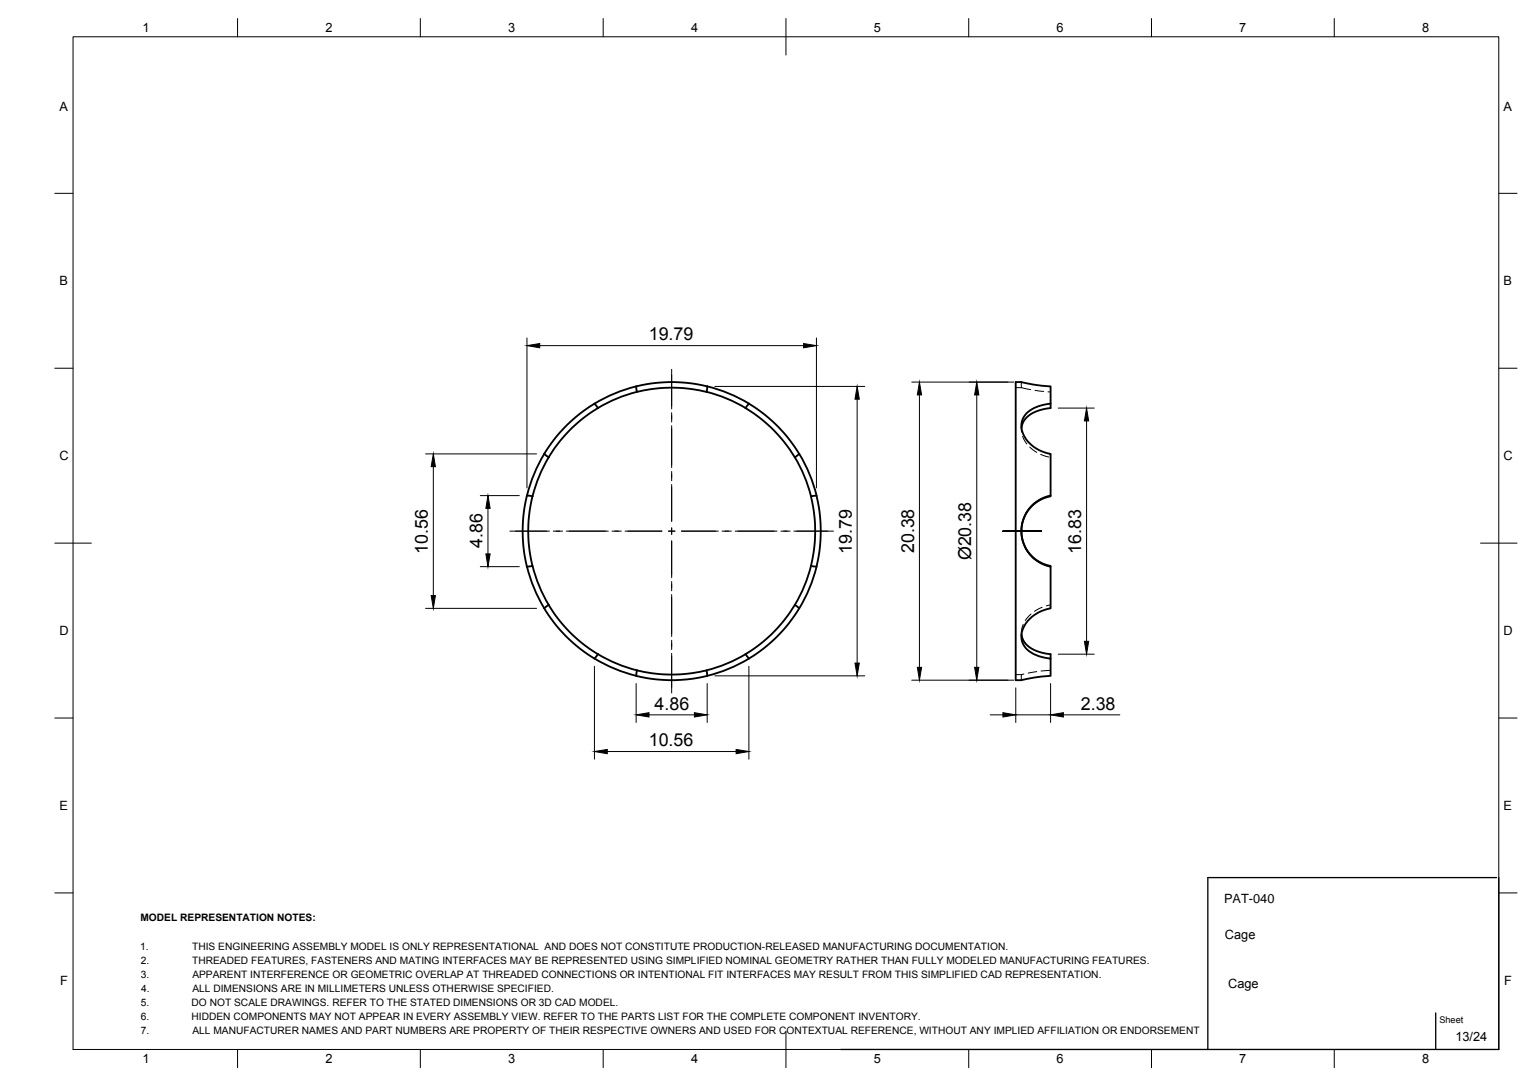
ISO-10303-21;
HEADER;
/* Generated by software containing ST-Developer
 * from STEP Tools, Inc. (www.steptools.com) 
 */

FILE_DESCRIPTION(
/* description */ ('Four-bar tabletop demonstrator'),
/* implementation_level */ '2;1');

FILE_NAME(
/* name */ 'Cage.step',
/* time_stamp */ '2026-10-29T17:05:23-07:00',
/* author */ (''),
/* organization */ (''),
/* preprocessor_version */ 'ST-DEVELOPER v20.2',
/* originating_system */ 'Autodesk Translation Framework v15.17.0.0',
/* authorisation */ '');

FILE_SCHEMA (('AUTOMOTIVE_DESIGN { 1 0 10303 214 3 1 1 }'));
ENDSEC;

DATA;
#10=MECHANICAL_DESIGN_GEOMETRIC_PRESENTATION_REPRESENTATION('',(#351),#6705);
#255=SPHERICAL_SURFACE('',#3806,0.247676);
#256=SPHERICAL_SURFACE('',#3822,0.247676);
#257=SPHERICAL_SURFACE('',#3827,0.247676);
#258=SPHERICAL_SURFACE('',#3832,0.247676);
#259=SPHERICAL_SURFACE('',#3837,0.247676);
#260=SPHERICAL_SURFACE('',#3842,0.247676);
#261=SPHERICAL_SURFACE('',#3847,0.247676);
#262=SPHERICAL_SURFACE('',#3855,0.247676);
#284=B_SPLINE_CURVE_WITH_KNOTS('',3,(#5773,#5774,#5775,#5776,#5777,#5778,
#5779,#5780,#5781,#5782,#5783,#5784,#5785,#5786,#5787,#5788,#5789,#5790,
#5791,#5792,#5793,#5794),.UNSPECIFIED.,.F.,.F.,(4,2,2,2,2,2,2,2,2,2,4),
(0.0473477652366656,0.126350602536658,0.189525903804987,0.252701205073317,
0.313298422430275,0.373895639787233,0.434492857144191,0.495090074501149,
0.558265375769478,0.621440677037807,0.7004435143378),.UNSPECIFIED.);
#285=B_SPLINE_CURVE_WITH_KNOTS('',3,(#5798,#5799,#5800,#5801,#5802,#5803,
#5804,#5805,#5806,#5807,#5808,#5809,#5810,#5811,#5812,#5813,#5814,#5815,
#5816,#5817,#5818,#5819),.UNSPECIFIED.,.F.,.F.,(4,2,2,2,2,2,2,2,2,2,4),
(0.0464897534940957,0.0852567806515119,0.170513561303024,0.246687263103517,
0.308657850341199,0.370628437578881,0.432599024816563,0.494569612054245,
0.570743313854739,0.656000094506251,0.694767121663666),.UNSPECIFIED.);
#286=B_SPLINE_CURVE_WITH_KNOTS('',3,(#5825,#5826,#5827,#5828,#5829,#5830,
#5831,#5832,#5833,#5834,#5835,#5836,#5837,#5838,#5839,#5840,#5841,#5842,
#5843,#5844,#5845,#5846),.UNSPECIFIED.,.F.,.F.,(4,2,2,2,2,2,2,2,2,2,4),
(0.0464897534940957,0.0852567806515118,0.170513561303024,0.246687263103517,
0.308657850341199,0.370628437578881,0.432599024816563,0.494569612054245,
0.570743313854738,0.65600009450625,0.694767121663666),.UNSPECIFIED.);
#287=B_SPLINE_CURVE_WITH_KNOTS('',3,(#5850,#5851,#5852,#5853,#5854,#5855,
#5856,#5857,#5858,#5859,#5860,#5861,#5862,#5863,#5864,#5865,#5866,#5867,
#5868,#5869,#5870,#5871),.UNSPECIFIED.,.F.,.F.,(4,2,2,2,2,2,2,2,2,2,4),
(0.0464897534940957,0.0852567806515119,0.170513561303024,0.246687263103517,
0.308657850341199,0.370628437578881,0.432599024816563,0.494569612054245,
0.570743313854739,0.656000094506251,0.694767121663666),.UNSPECIFIED.);
#288=B_SPLINE_CURVE_WITH_KNOTS('',3,(#5875,#5876,#5877,#5878,#5879,#5880,
#5881,#5882,#5883,#5884,#5885,#5886),.UNSPECIFIED.,.F.,.F.,(4,2,2,2,2,4),
(0.0464897534940957,0.0852567806515119,0.170513561303024,0.246687263103517,
0.308657850341199,0.370628437578881),.UNSPECIFIED.);
#289=B_SPLINE_CURVE_WITH_KNOTS('',3,(#5891,#5892,#5893,#5894,#5895,#5896,
#5897,#5898,#5899,#5900,#5901,#5902),.UNSPECIFIED.,.F.,.F.,(4,2,2,2,2,4),
(0.370628437578881,0.432599024816563,0.494569612054245,0.570743313854738,
0.65600009450625,0.694767121663666),.UNSPECIFIED.);
#290=B_SPLINE_CURVE_WITH_KNOTS('',3,(#5906,#5907,#5908,#5909,#5910,#5911,
#5912,#5913,#5914,#5915,#5916,#5917,#5918,#5919,#5920,#5921,#5922,#5923,
#5924,#5925,#5926,#5927),.UNSPECIFIED.,.F.,.F.,(4,2,2,2,2,2,2,2,2,2,4),
(0.0464897534940957,0.0852567806515121,0.170513561303024,0.246687263103518,
0.308657850341199,0.370628437578881,0.432599024816563,0.494569612054245,
0.570743313854738,0.65600009450625,0.694767121663666),.UNSPECIFIED.);
#291=B_SPLINE_CURVE_WITH_KNOTS('',3,(#5931,#5932,#5933,#5934,#5935,#5936,
#5937,#5938,#5939,#5940,#5941,#5942,#5943,#5944,#5945,#5946,#5947,#5948,
#5949,#5950,#5951,#5952),.UNSPECIFIED.,.F.,.F.,(4,2,2,2,2,2,2,2,2,2,4),
(0.0464897534940957,0.0852567806515119,0.170513561303024,0.246687263103517,
0.308657850341199,0.370628437578881,0.432599024816563,0.494569612054245,
0.570743313854738,0.65600009450625,0.694767121663667),.UNSPECIFIED.);
#292=B_SPLINE_CURVE_WITH_KNOTS('',3,(#5956,#5957,#5958,#5959,#5960,#5961,
#5962,#5963,#5964,#5965,#5966,#5967,#5968,#5969,#5970,#5971,#5972,#5973,
#5974,#5975,#5976,#5977),.UNSPECIFIED.,.F.,.F.,(4,2,2,2,2,2,2,2,2,2,4),
(0.0464897534940957,0.0852567806515119,0.170513561303024,0.246687263103517,
0.308657850341199,0.370628437578881,0.432599024816563,0.494569612054245,
0.570743313854738,0.65600009450625,0.694767121663666),.UNSPECIFIED.);
#293=B_SPLINE_CURVE_WITH_KNOTS('',3,(#5981,#5982,#5983,#5984,#5985,#5986,
#5987,#5988,#5989,#5990,#5991,#5992,#5993,#5994,#5995,#5996,#5997,#5998,
#5999,#6000,#6001,#6002),.UNSPECIFIED.,.F.,.F.,(4,2,2,2,2,2,2,2,2,2,4),
(0.0464897534940957,0.0852567806515119,0.170513561303024,0.246687263103517,
0.308657850341199,0.370628437578881,0.432599024816563,0.494569612054245,
0.570743313854739,0.656000094506251,0.694767121663667),.UNSPECIFIED.);
#294=B_SPLINE_CURVE_WITH_KNOTS('',3,(#6010,#6011,#6012,#6013,#6014,#6015,
#6016,#6017,#6018,#6019,#6020,#6021,#6022,#6023,#6024,#6025,#6026,#6027,
#6028,#6029,#6030,#6031),.UNSPECIFIED.,.F.,.F.,(4,2,2,2,2,2,2,2,2,2,4),
(0.0473477652366656,0.126350602536658,0.189525903804987,0.252701205073316,
0.313298422430274,0.373895639787232,0.434492857144191,0.495090074501149,
0.558265375769478,0.621440677037807,0.7004435143378),.UNSPECIFIED.);
#295=B_SPLINE_CURVE_WITH_KNOTS('',3,(#6039,#6040,#6041,#6042,#6043,#6044,
#6045,#6046,#6047,#6048,#6049,#6050,#6051,#6052,#6053,#6054,#6055,#6056,
#6057,#6058,#6059,#6060),.UNSPECIFIED.,.F.,.F.,(4,2,2,2,2,2,2,2,2,2,4),
(0.0473477652366656,0.126350602536658,0.189525903804987,0.252701205073317,
0.313298422430275,0.373895639787233,0.434492857144191,0.495090074501149,
0.558265375769478,0.621440677037807,0.7004435143378),.UNSPECIFIED.);
#296=B_SPLINE_CURVE_WITH_KNOTS('',3,(#6069,#6070,#6071,#6072,#6073,#6074,
#6075,#6076,#6077,#6078,#6079,#6080),.UNSPECIFIED.,.F.,.F.,(4,2,2,2,2,4),
(0.0473477652366656,0.126350602536658,0.189525903804987,0.252701205073316,
0.313298422430275,0.373895639787233),.UNSPECIFIED.);
#297=B_SPLINE_CURVE_WITH_KNOTS('',3,(#6082,#6083,#6084,#6085,#6086,#6087,
#6088,#6089,#6090,#6091,#6092,#6093),.UNSPECIFIED.,.F.,.F.,(4,2,2,2,2,4),
(0.373895639787233,0.434492857144191,0.495090074501149,0.558265375769478,
0.621440677037807,0.7004435143378),.UNSPECIFIED.);
#298=B_SPLINE_CURVE_WITH_KNOTS('',3,(#6100,#6101,#6102,#6103,#6104,#6105,
#6106,#6107,#6108,#6109,#6110,#6111,#6112,#6113,#6114,#6115,#6116,#6117,
#6118,#6119,#6120,#6121),.UNSPECIFIED.,.F.,.F.,(4,2,2,2,2,2,2,2,2,2,4),
(0.0473477652366656,0.126350602536658,0.189525903804987,0.252701205073316,
0.313298422430275,0.373895639787233,0.434492857144191,0.495090074501149,
0.558265375769478,0.621440677037807,0.7004435143378),.UNSPECIFIED.);
#299=B_SPLINE_CURVE_WITH_KNOTS('',3,(#6129,#6130,#6131,#6132,#6133,#6134,
#6135,#6136,#6137,#6138,#6139,#6140,#6141,#6142,#6143,#6144,#6145,#6146,
#6147,#6148,#6149,#6150),.UNSPECIFIED.,.F.,.F.,(4,2,2,2,2,2,2,2,2,2,4),
(0.0473477652366656,0.126350602536658,0.189525903804987,0.252701205073317,
0.313298422430275,0.373895639787233,0.434492857144191,0.495090074501149,
0.558265375769478,0.621440677037807,0.7004435143378),.UNSPECIFIED.);
#300=B_SPLINE_CURVE_WITH_KNOTS('',3,(#6158,#6159,#6160,#6161,#6162,#6163,
#6164,#6165,#6166,#6167,#6168,#6169,#6170,#6171,#6172,#6173,#6174,#6175,
#6176,#6177,#6178,#6179),.UNSPECIFIED.,.F.,.F.,(4,2,2,2,2,2,2,2,2,2,4),
(0.0473477652366656,0.126350602536658,0.189525903804987,0.252701205073316,
0.313298422430275,0.373895639787233,0.434492857144191,0.495090074501149,
0.558265375769478,0.621440677037807,0.7004435143378),.UNSPECIFIED.);
#301=B_SPLINE_CURVE_WITH_KNOTS('',3,(#6188,#6189,#6190,#6191,#6192,#6193,
#6194,#6195,#6196,#6197,#6198,#6199,#6200,#6201,#6202,#6203,#6204,#6205,
#6206,#6207,#6208,#6209),.UNSPECIFIED.,.F.,.F.,(4,2,2,2,2,2,2,2,2,2,4),
(0.0473477652366656,0.126350602536658,0.189525903804987,0.252701205073317,
0.313298422430275,0.373895639787233,0.434492857144191,0.495090074501149,
0.558265375769478,0.621440677037807,0.7004435143378),.UNSPECIFIED.);
#314=SHAPE_REPRESENTATION_RELATIONSHIP('SRR','None',#6823,#329);
#329=ADVANCED_BREP_SHAPE_REPRESENTATION('',(#373),#6696);
#351=STYLED_ITEM('',(#6989),#373);
#373=MANIFOLD_SOLID_BREP('Continuous crown cage',#3396);
#430=FACE_BOUND('',#938,.T.);
#508=PLANE('',#3819);
#509=PLANE('',#3824);
#510=PLANE('',#3829);
#511=PLANE('',#3834);
#512=PLANE('',#3839);
#513=PLANE('',#3844);
#514=PLANE('',#3853);
#515=PLANE('',#3857);
#516=PLANE('',#3858);
#668=FACE_OUTER_BOUND('',#920,.T.);
#669=FACE_OUTER_BOUND('',#921,.T.);
#670=FACE_OUTER_BOUND('',#922,.T.);
#671=FACE_OUTER_BOUND('',#923,.T.);
#672=FACE_OUTER_BOUND('',#924,.T.);
#673=FACE_OUTER_BOUND('',#925,.T.);
#674=FACE_OUTER_BOUND('',#926,.T.);
#675=FACE_OUTER_BOUND('',#927,.T.);
#676=FACE_OUTER_BOUND('',#928,.T.);
#677=FACE_OUTER_BOUND('',#929,.T.);
#678=FACE_OUTER_BOUND('',#930,.T.);
#679=FACE_OUTER_BOUND('',#931,.T.);
#680=FACE_OUTER_BOUND('',#932,.T.);
#681=FACE_OUTER_BOUND('',#933,.T.);
#682=FACE_OUTER_BOUND('',#934,.T.);
#683=FACE_OUTER_BOUND('',#935,.T.);
#684=FACE_OUTER_BOUND('',#936,.T.);
#685=FACE_OUTER_BOUND('',#937,.T.);
#686=FACE_OUTER_BOUND('',#939,.T.);
#920=EDGE_LOOP('',(#2708,#2709,#2710,#2711));
#921=EDGE_LOOP('',(#2712,#2713,#2714,#2715,#2716,#2717,#2718,#2719,#2720,
#2721,#2722,#2723,#2724,#2725,#2726,#2727,#2728,#2729,#2730,#2731));
#922=EDGE_LOOP('',(#2732,#2733,#2734,#2735));
#923=EDGE_LOOP('',(#2736,#2737,#2738,#2739));
#924=EDGE_LOOP('',(#2740,#2741,#2742,#2743));
#925=EDGE_LOOP('',(#2744,#2745,#2746,#2747));
#926=EDGE_LOOP('',(#2748,#2749,#2750,#2751));
#927=EDGE_LOOP('',(#2752,#2753,#2754,#2755,#2756,#2757));
#928=EDGE_LOOP('',(#2758,#2759,#2760,#2761));
#929=EDGE_LOOP('',(#2762,#2763,#2764,#2765));
#930=EDGE_LOOP('',(#2766,#2767,#2768,#2769));
#931=EDGE_LOOP('',(#2770,#2771,#2772,#2773));
#932=EDGE_LOOP('',(#2774,#2775,#2776,#2777));
#933=EDGE_LOOP('',(#2778,#2779,#2780,#2781));
#934=EDGE_LOOP('',(#2782,#2783,#2784,#2785,#2786,#2787,#2788,#2789,#2790,
#2791,#2792,#2793,#2794,#2795,#2796,#2797,#2798,#2799,#2800,#2801));
#935=EDGE_LOOP('',(#2802,#2803,#2804,#2805));
#936=EDGE_LOOP('',(#2806,#2807,#2808,#2809));
#937=EDGE_LOOP('',(#2810));
#938=EDGE_LOOP('',(#2811));
#939=EDGE_LOOP('',(#2812,#2813,#2814,#2815));
#1140=LINE('',#5888,#1310);
#1141=LINE('',#6184,#1311);
#1310=VECTOR('',#4639,1.019052);
#1311=VECTOR('',#4716,0.980948);
#1504=CIRCLE('',#3807,0.243053047864041);
#1505=CIRCLE('',#3808,0.243053047864041);
#1506=CIRCLE('',#3810,1.019052);
#1507=CIRCLE('',#3811,1.019052);
#1508=CIRCLE('',#3812,1.019052);
#1509=CIRCLE('',#3813,1.019052);
#1510=CIRCLE('',#3814,1.019052);
#1511=CIRCLE('',#3815,1.019052);
#1512=CIRCLE('',#3816,1.019052);
#1513=CIRCLE('',#3817,1.019052);
#1514=CIRCLE('',#3818,1.019052);
#1515=CIRCLE('',#3820,0.980948);
#1516=CIRCLE('',#3821,0.243053047864041);
#1517=CIRCLE('',#3823,0.243053047864041);
#1518=CIRCLE('',#3825,0.980948);
#1519=CIRCLE('',#3826,0.243053047864041);
#1520=CIRCLE('',#3828,0.243053047864041);
#1521=CIRCLE('',#3830,0.980948);
#1522=CIRCLE('',#3831,0.243053047864041);
#1523=CIRCLE('',#3833,0.243053047864041);
#1524=CIRCLE('',#3835,0.980948);
#1525=CIRCLE('',#3836,0.243053047864041);
#1526=CIRCLE('',#3838,0.243053047864041);
#1527=CIRCLE('',#3840,0.980948);
#1528=CIRCLE('',#3841,0.243053047864041);
#1529=CIRCLE('',#3843,0.243053047864041);
#1530=CIRCLE('',#3845,0.980948);
#1531=CIRCLE('',#3846,0.243053047864041);
#1532=CIRCLE('',#3848,0.243053047864041);
#1533=CIRCLE('',#3850,0.980948);
#1534=CIRCLE('',#3851,0.980948);
#1535=CIRCLE('',#3852,0.980948);
#1536=CIRCLE('',#3854,0.243053047864041);
#1537=CIRCLE('',#3856,0.243053047864041);
#1749=VERTEX_POINT('',#5771);
#1750=VERTEX_POINT('',#5772);
#1751=VERTEX_POINT('',#5795);
#1752=VERTEX_POINT('',#5797);
#1753=VERTEX_POINT('',#5822);
#1754=VERTEX_POINT('',#5824);
#1755=VERTEX_POINT('',#5847);
#1756=VERTEX_POINT('',#5849);
#1757=VERTEX_POINT('',#5872);
#1758=VERTEX_POINT('',#5874);
#1759=VERTEX_POINT('',#5887);
#1760=VERTEX_POINT('',#5890);
#1761=VERTEX_POINT('',#5903);
#1762=VERTEX_POINT('',#5905);
#1763=VERTEX_POINT('',#5928);
#1764=VERTEX_POINT('',#5930);
#1765=VERTEX_POINT('',#5953);
#1766=VERTEX_POINT('',#5955);
#1767=VERTEX_POINT('',#5978);
#1768=VERTEX_POINT('',#5980);
#1769=VERTEX_POINT('',#6005);
#1770=VERTEX_POINT('',#6009);
#1771=VERTEX_POINT('',#6034);
#1772=VERTEX_POINT('',#6038);
#1773=VERTEX_POINT('',#6063);
#1774=VERTEX_POINT('',#6067);
#1775=VERTEX_POINT('',#6068);
#1776=VERTEX_POINT('',#6095);
#1777=VERTEX_POINT('',#6099);
#1778=VERTEX_POINT('',#6124);
#1779=VERTEX_POINT('',#6128);
#1780=VERTEX_POINT('',#6153);
#1781=VERTEX_POINT('',#6157);
#1782=VERTEX_POINT('',#6182);
#1783=VERTEX_POINT('',#6185);
#1784=VERTEX_POINT('',#6187);
#2090=EDGE_CURVE('',#1749,#1750,#284,.T.);
#2091=EDGE_CURVE('',#1751,#1749,#1504,.T.);
#2092=EDGE_CURVE('',#1752,#1751,#285,.T.);
#2093=EDGE_CURVE('',#1750,#1752,#1505,.T.);
#2094=EDGE_CURVE('',#1753,#1751,#1506,.T.);
#2095=EDGE_CURVE('',#1753,#1754,#286,.T.);
#2096=EDGE_CURVE('',#1755,#1754,#1507,.T.);
#2097=EDGE_CURVE('',#1755,#1756,#287,.T.);
#2098=EDGE_CURVE('',#1757,#1756,#1508,.T.);
#2099=EDGE_CURVE('',#1757,#1758,#288,.T.);
#2100=EDGE_CURVE('',#1758,#1759,#1140,.T.);
#2101=EDGE_CURVE('',#1759,#1759,#1509,.T.);
#2102=EDGE_CURVE('',#1758,#1760,#289,.T.);
#2103=EDGE_CURVE('',#1761,#1760,#1510,.T.);
#2104=EDGE_CURVE('',#1761,#1762,#290,.T.);
#2105=EDGE_CURVE('',#1763,#1762,#1511,.T.);
#2106=EDGE_CURVE('',#1763,#1764,#291,.T.);
#2107=EDGE_CURVE('',#1765,#1764,#1512,.T.);
#2108=EDGE_CURVE('',#1765,#1766,#292,.T.);
#2109=EDGE_CURVE('',#1767,#1766,#1513,.T.);
#2110=EDGE_CURVE('',#1767,#1768,#293,.T.);
#2111=EDGE_CURVE('',#1752,#1768,#1514,.T.);
#2112=EDGE_CURVE('',#1749,#1769,#1515,.T.);
#2113=EDGE_CURVE('',#1769,#1753,#1516,.T.);
#2114=EDGE_CURVE('',#1770,#1769,#294,.T.);
#2115=EDGE_CURVE('',#1754,#1770,#1517,.T.);
#2116=EDGE_CURVE('',#1770,#1771,#1518,.T.);
#2117=EDGE_CURVE('',#1771,#1755,#1519,.T.);
#2118=EDGE_CURVE('',#1772,#1771,#295,.T.);
#2119=EDGE_CURVE('',#1756,#1772,#1520,.T.);
#2120=EDGE_CURVE('',#1772,#1773,#1521,.T.);
#2121=EDGE_CURVE('',#1773,#1757,#1522,.T.);
#2122=EDGE_CURVE('',#1774,#1775,#296,.T.);
#2123=EDGE_CURVE('',#1760,#1774,#1523,.T.);
#2124=EDGE_CURVE('',#1775,#1773,#297,.T.);
#2125=EDGE_CURVE('',#1774,#1776,#1524,.T.);
#2126=EDGE_CURVE('',#1776,#1761,#1525,.T.);
#2127=EDGE_CURVE('',#1777,#1776,#298,.T.);
#2128=EDGE_CURVE('',#1762,#1777,#1526,.T.);
#2129=EDGE_CURVE('',#1777,#1778,#1527,.T.);
#2130=EDGE_CURVE('',#1778,#1763,#1528,.T.);
#2131=EDGE_CURVE('',#1779,#1778,#299,.T.);
#2132=EDGE_CURVE('',#1764,#1779,#1529,.T.);
#2133=EDGE_CURVE('',#1779,#1780,#1530,.T.);
#2134=EDGE_CURVE('',#1780,#1765,#1531,.T.);
#2135=EDGE_CURVE('',#1781,#1780,#300,.T.);
#2136=EDGE_CURVE('',#1766,#1781,#1532,.T.);
#2137=EDGE_CURVE('',#1782,#1782,#1533,.T.);
#2138=EDGE_CURVE('',#1782,#1775,#1141,.T.);
#2139=EDGE_CURVE('',#1783,#1750,#1534,.T.);
#2140=EDGE_CURVE('',#1783,#1784,#301,.T.);
#2141=EDGE_CURVE('',#1781,#1784,#1535,.T.);
#2142=EDGE_CURVE('',#1768,#1783,#1536,.T.);
#2143=EDGE_CURVE('',#1784,#1767,#1537,.T.);
#2708=ORIENTED_EDGE('',*,*,#2090,.F.);
#2709=ORIENTED_EDGE('',*,*,#2091,.F.);
#2710=ORIENTED_EDGE('',*,*,#2092,.F.);
#2711=ORIENTED_EDGE('',*,*,#2093,.F.);
#2712=ORIENTED_EDGE('',*,*,#2092,.T.);
#2713=ORIENTED_EDGE('',*,*,#2094,.F.);
#2714=ORIENTED_EDGE('',*,*,#2095,.T.);
#2715=ORIENTED_EDGE('',*,*,#2096,.F.);
#2716=ORIENTED_EDGE('',*,*,#2097,.T.);
#2717=ORIENTED_EDGE('',*,*,#2098,.F.);
#2718=ORIENTED_EDGE('',*,*,#2099,.T.);
#2719=ORIENTED_EDGE('',*,*,#2100,.T.);
#2720=ORIENTED_EDGE('',*,*,#2101,.F.);
#2721=ORIENTED_EDGE('',*,*,#2100,.F.);
#2722=ORIENTED_EDGE('',*,*,#2102,.T.);
#2723=ORIENTED_EDGE('',*,*,#2103,.F.);
#2724=ORIENTED_EDGE('',*,*,#2104,.T.);
#2725=ORIENTED_EDGE('',*,*,#2105,.F.);
#2726=ORIENTED_EDGE('',*,*,#2106,.T.);
#2727=ORIENTED_EDGE('',*,*,#2107,.F.);
#2728=ORIENTED_EDGE('',*,*,#2108,.T.);
#2729=ORIENTED_EDGE('',*,*,#2109,.F.);
#2730=ORIENTED_EDGE('',*,*,#2110,.T.);
#2731=ORIENTED_EDGE('',*,*,#2111,.F.);
#2732=ORIENTED_EDGE('',*,*,#2091,.T.);
#2733=ORIENTED_EDGE('',*,*,#2112,.T.);
#2734=ORIENTED_EDGE('',*,*,#2113,.T.);
#2735=ORIENTED_EDGE('',*,*,#2094,.T.);
#2736=ORIENTED_EDGE('',*,*,#2114,.F.);
#2737=ORIENTED_EDGE('',*,*,#2115,.F.);
#2738=ORIENTED_EDGE('',*,*,#2095,.F.);
#2739=ORIENTED_EDGE('',*,*,#2113,.F.);
#2740=ORIENTED_EDGE('',*,*,#2115,.T.);
#2741=ORIENTED_EDGE('',*,*,#2116,.T.);
#2742=ORIENTED_EDGE('',*,*,#2117,.T.);
#2743=ORIENTED_EDGE('',*,*,#2096,.T.);
#2744=ORIENTED_EDGE('',*,*,#2118,.F.);
#2745=ORIENTED_EDGE('',*,*,#2119,.F.);
#2746=ORIENTED_EDGE('',*,*,#2097,.F.);
#2747=ORIENTED_EDGE('',*,*,#2117,.F.);
#2748=ORIENTED_EDGE('',*,*,#2119,.T.);
#2749=ORIENTED_EDGE('',*,*,#2120,.T.);
#2750=ORIENTED_EDGE('',*,*,#2121,.T.);
#2751=ORIENTED_EDGE('',*,*,#2098,.T.);
#2752=ORIENTED_EDGE('',*,*,#2122,.F.);
#2753=ORIENTED_EDGE('',*,*,#2123,.F.);
#2754=ORIENTED_EDGE('',*,*,#2102,.F.);
#2755=ORIENTED_EDGE('',*,*,#2099,.F.);
#2756=ORIENTED_EDGE('',*,*,#2121,.F.);
#2757=ORIENTED_EDGE('',*,*,#2124,.F.);
#2758=ORIENTED_EDGE('',*,*,#2123,.T.);
#2759=ORIENTED_EDGE('',*,*,#2125,.T.);
#2760=ORIENTED_EDGE('',*,*,#2126,.T.);
#2761=ORIENTED_EDGE('',*,*,#2103,.T.);
#2762=ORIENTED_EDGE('',*,*,#2127,.F.);
#2763=ORIENTED_EDGE('',*,*,#2128,.F.);
#2764=ORIENTED_EDGE('',*,*,#2104,.F.);
#2765=ORIENTED_EDGE('',*,*,#2126,.F.);
#2766=ORIENTED_EDGE('',*,*,#2128,.T.);
#2767=ORIENTED_EDGE('',*,*,#2129,.T.);
#2768=ORIENTED_EDGE('',*,*,#2130,.T.);
#2769=ORIENTED_EDGE('',*,*,#2105,.T.);
#2770=ORIENTED_EDGE('',*,*,#2131,.F.);
#2771=ORIENTED_EDGE('',*,*,#2132,.F.);
#2772=ORIENTED_EDGE('',*,*,#2106,.F.);
#2773=ORIENTED_EDGE('',*,*,#2130,.F.);
#2774=ORIENTED_EDGE('',*,*,#2132,.T.);
#2775=ORIENTED_EDGE('',*,*,#2133,.T.);
#2776=ORIENTED_EDGE('',*,*,#2134,.T.);
#2777=ORIENTED_EDGE('',*,*,#2107,.T.);
#2778=ORIENTED_EDGE('',*,*,#2108,.F.);
#2779=ORIENTED_EDGE('',*,*,#2134,.F.);
#2780=ORIENTED_EDGE('',*,*,#2135,.F.);
#2781=ORIENTED_EDGE('',*,*,#2136,.F.);
#2782=ORIENTED_EDGE('',*,*,#2137,.F.);
#2783=ORIENTED_EDGE('',*,*,#2138,.T.);
#2784=ORIENTED_EDGE('',*,*,#2124,.T.);
#2785=ORIENTED_EDGE('',*,*,#2120,.F.);
#2786=ORIENTED_EDGE('',*,*,#2118,.T.);
#2787=ORIENTED_EDGE('',*,*,#2116,.F.);
#2788=ORIENTED_EDGE('',*,*,#2114,.T.);
#2789=ORIENTED_EDGE('',*,*,#2112,.F.);
#2790=ORIENTED_EDGE('',*,*,#2090,.T.);
#2791=ORIENTED_EDGE('',*,*,#2139,.F.);
#2792=ORIENTED_EDGE('',*,*,#2140,.T.);
#2793=ORIENTED_EDGE('',*,*,#2141,.F.);
#2794=ORIENTED_EDGE('',*,*,#2135,.T.);
#2795=ORIENTED_EDGE('',*,*,#2133,.F.);
#2796=ORIENTED_EDGE('',*,*,#2131,.T.);
#2797=ORIENTED_EDGE('',*,*,#2129,.F.);
#2798=ORIENTED_EDGE('',*,*,#2127,.T.);
#2799=ORIENTED_EDGE('',*,*,#2125,.F.);
#2800=ORIENTED_EDGE('',*,*,#2122,.T.);
#2801=ORIENTED_EDGE('',*,*,#2138,.F.);
#2802=ORIENTED_EDGE('',*,*,#2093,.T.);
#2803=ORIENTED_EDGE('',*,*,#2111,.T.);
#2804=ORIENTED_EDGE('',*,*,#2142,.T.);
#2805=ORIENTED_EDGE('',*,*,#2139,.T.);
#2806=ORIENTED_EDGE('',*,*,#2110,.F.);
#2807=ORIENTED_EDGE('',*,*,#2143,.F.);
#2808=ORIENTED_EDGE('',*,*,#2140,.F.);
#2809=ORIENTED_EDGE('',*,*,#2142,.F.);
#2810=ORIENTED_EDGE('',*,*,#2101,.T.);
#2811=ORIENTED_EDGE('',*,*,#2137,.T.);
#2812=ORIENTED_EDGE('',*,*,#2136,.T.);
#2813=ORIENTED_EDGE('',*,*,#2141,.T.);
#2814=ORIENTED_EDGE('',*,*,#2143,.T.);
#2815=ORIENTED_EDGE('',*,*,#2109,.T.);
#3147=CYLINDRICAL_SURFACE('',#3809,1.019052);
#3148=CYLINDRICAL_SURFACE('',#3849,0.980948);
#3284=ADVANCED_FACE('',(#668),#255,.F.);
#3285=ADVANCED_FACE('',(#669),#3147,.T.);
#3286=ADVANCED_FACE('',(#670),#508,.T.);
#3287=ADVANCED_FACE('',(#671),#256,.F.);
#3288=ADVANCED_FACE('',(#672),#509,.T.);
#3289=ADVANCED_FACE('',(#673),#257,.F.);
#3290=ADVANCED_FACE('',(#674),#510,.T.);
#3291=ADVANCED_FACE('',(#675),#258,.F.);
#3292=ADVANCED_FACE('',(#676),#511,.T.);
#3293=ADVANCED_FACE('',(#677),#259,.F.);
#3294=ADVANCED_FACE('',(#678),#512,.T.);
#3295=ADVANCED_FACE('',(#679),#260,.F.);
#3296=ADVANCED_FACE('',(#680),#513,.T.);
#3297=ADVANCED_FACE('',(#681),#261,.F.);
#3298=ADVANCED_FACE('',(#682),#3148,.F.);
#3299=ADVANCED_FACE('',(#683),#514,.T.);
#3300=ADVANCED_FACE('',(#684),#262,.F.);
#3301=ADVANCED_FACE('',(#685,#430),#515,.T.);
#3302=ADVANCED_FACE('',(#686),#516,.T.);
#3396=CLOSED_SHELL('',(#3284,#3285,#3286,#3287,#3288,#3289,#3290,#3291,
#3292,#3293,#3294,#3295,#3296,#3297,#3298,#3299,#3300,#3301,#3302));
#3805=AXIS2_PLACEMENT_3D('',#5769,#4623,#4624);
#3806=AXIS2_PLACEMENT_3D('',#5770,#4625,#4626);
#3807=AXIS2_PLACEMENT_3D('',#5796,#4627,#4628);
#3808=AXIS2_PLACEMENT_3D('',#5820,#4629,#4630);
#3809=AXIS2_PLACEMENT_3D('',#5821,#4631,#4632);
#3810=AXIS2_PLACEMENT_3D('',#5823,#4633,#4634);
#3811=AXIS2_PLACEMENT_3D('',#5848,#4635,#4636);
#3812=AXIS2_PLACEMENT_3D('',#5873,#4637,#4638);
#3813=AXIS2_PLACEMENT_3D('',#5889,#4640,#4641);
#3814=AXIS2_PLACEMENT_3D('',#5904,#4642,#4643);
#3815=AXIS2_PLACEMENT_3D('',#5929,#4644,#4645);
#3816=AXIS2_PLACEMENT_3D('',#5954,#4646,#4647);
#3817=AXIS2_PLACEMENT_3D('',#5979,#4648,#4649);
#3818=AXIS2_PLACEMENT_3D('',#6003,#4650,#4651);
#3819=AXIS2_PLACEMENT_3D('',#6004,#4652,#4653);
#3820=AXIS2_PLACEMENT_3D('',#6006,#4654,#4655);
#3821=AXIS2_PLACEMENT_3D('',#6007,#4656,#4657);
#3822=AXIS2_PLACEMENT_3D('',#6008,#4658,#4659);
#3823=AXIS2_PLACEMENT_3D('',#6032,#4660,#4661);
#3824=AXIS2_PLACEMENT_3D('',#6033,#4662,#4663);
#3825=AXIS2_PLACEMENT_3D('',#6035,#4664,#4665);
#3826=AXIS2_PLACEMENT_3D('',#6036,#4666,#4667);
#3827=AXIS2_PLACEMENT_3D('',#6037,#4668,#4669);
#3828=AXIS2_PLACEMENT_3D('',#6061,#4670,#4671);
#3829=AXIS2_PLACEMENT_3D('',#6062,#4672,#4673);
#3830=AXIS2_PLACEMENT_3D('',#6064,#4674,#4675);
#3831=AXIS2_PLACEMENT_3D('',#6065,#4676,#4677);
#3832=AXIS2_PLACEMENT_3D('',#6066,#4678,#4679);
#3833=AXIS2_PLACEMENT_3D('',#6081,#4680,#4681);
#3834=AXIS2_PLACEMENT_3D('',#6094,#4682,#4683);
#3835=AXIS2_PLACEMENT_3D('',#6096,#4684,#4685);
#3836=AXIS2_PLACEMENT_3D('',#6097,#4686,#4687);
#3837=AXIS2_PLACEMENT_3D('',#6098,#4688,#4689);
#3838=AXIS2_PLACEMENT_3D('',#6122,#4690,#4691);
#3839=AXIS2_PLACEMENT_3D('',#6123,#4692,#4693);
#3840=AXIS2_PLACEMENT_3D('',#6125,#4694,#4695);
#3841=AXIS2_PLACEMENT_3D('',#6126,#4696,#4697);
#3842=AXIS2_PLACEMENT_3D('',#6127,#4698,#4699);
#3843=AXIS2_PLACEMENT_3D('',#6151,#4700,#4701);
#3844=AXIS2_PLACEMENT_3D('',#6152,#4702,#4703);
#3845=AXIS2_PLACEMENT_3D('',#6154,#4704,#4705);
#3846=AXIS2_PLACEMENT_3D('',#6155,#4706,#4707);
#3847=AXIS2_PLACEMENT_3D('',#6156,#4708,#4709);
#3848=AXIS2_PLACEMENT_3D('',#6180,#4710,#4711);
#3849=AXIS2_PLACEMENT_3D('',#6181,#4712,#4713);
#3850=AXIS2_PLACEMENT_3D('',#6183,#4714,#4715);
#3851=AXIS2_PLACEMENT_3D('',#6186,#4717,#4718);
#3852=AXIS2_PLACEMENT_3D('',#6210,#4719,#4720);
#3853=AXIS2_PLACEMENT_3D('',#6211,#4721,#4722);
#3854=AXIS2_PLACEMENT_3D('',#6212,#4723,#4724);
#3855=AXIS2_PLACEMENT_3D('',#6213,#4725,#4726);
#3856=AXIS2_PLACEMENT_3D('',#6214,#4727,#4728);
#3857=AXIS2_PLACEMENT_3D('',#6215,#4729,#4730);
#3858=AXIS2_PLACEMENT_3D('',#6216,#4731,#4732);
#4623=DIRECTION('axis',(0.,0.,1.));
#4624=DIRECTION('refdir',(1.,0.,0.));
#4625=DIRECTION('center_axis',(0.,0.,1.));
#4626=DIRECTION('ref_axis',(1.,0.,0.));
#4627=DIRECTION('center_axis',(0.,-1.,0.));
#4628=DIRECTION('ref_axis',(0.,0.,-1.));
#4629=DIRECTION('center_axis',(0.,-1.,0.));
#4630=DIRECTION('ref_axis',(0.,0.,-1.));
#4631=DIRECTION('center_axis',(0.,1.,0.));
#4632=DIRECTION('ref_axis',(1.,0.,0.));
#4633=DIRECTION('center_axis',(0.,1.,0.));
#4634=DIRECTION('ref_axis',(1.,0.,0.));
#4635=DIRECTION('center_axis',(0.,1.,0.));
#4636=DIRECTION('ref_axis',(1.,0.,0.));
#4637=DIRECTION('center_axis',(0.,1.,0.));
#4638=DIRECTION('ref_axis',(1.,0.,0.));
#4639=DIRECTION('',(0.,-1.,0.));
#4640=DIRECTION('center_axis',(0.,-1.,0.));
#4641=DIRECTION('ref_axis',(1.,0.,0.));
#4642=DIRECTION('center_axis',(0.,1.,0.));
#4643=DIRECTION('ref_axis',(1.,0.,0.));
#4644=DIRECTION('center_axis',(0.,1.,0.));
#4645=DIRECTION('ref_axis',(1.,0.,0.));
#4646=DIRECTION('center_axis',(0.,1.,0.));
#4647=DIRECTION('ref_axis',(1.,0.,0.));
#4648=DIRECTION('center_axis',(0.,1.,0.));
#4649=DIRECTION('ref_axis',(1.,0.,0.));
#4650=DIRECTION('center_axis',(0.,1.,0.));
#4651=DIRECTION('ref_axis',(1.,0.,0.));
#4652=DIRECTION('center_axis',(0.,1.,0.));
#4653=DIRECTION('ref_axis',(1.,0.,0.));
#4654=DIRECTION('center_axis',(0.,-1.,0.));
#4655=DIRECTION('ref_axis',(1.,0.,0.));
#4656=DIRECTION('center_axis',(0.,-1.,0.));
#4657=DIRECTION('ref_axis',(0.,0.,-1.));
#4658=DIRECTION('center_axis',(6.12323399573677E-17,0.,1.));
#4659=DIRECTION('ref_axis',(1.,0.,0.));
#4660=DIRECTION('center_axis',(0.,-1.,0.));
#4661=DIRECTION('ref_axis',(0.,0.,-1.));
#4662=DIRECTION('center_axis',(0.,1.,0.));
#4663=DIRECTION('ref_axis',(1.,0.,0.));
#4664=DIRECTION('center_axis',(0.,-1.,0.));
#4665=DIRECTION('ref_axis',(1.,0.,0.));
#4666=DIRECTION('center_axis',(0.,-1.,0.));
#4667=DIRECTION('ref_axis',(0.,0.,-1.));
#4668=DIRECTION('center_axis',(0.,0.,1.));
#4669=DIRECTION('ref_axis',(1.,0.,0.));
#4670=DIRECTION('center_axis',(0.,-1.,0.));
#4671=DIRECTION('ref_axis',(0.,0.,-1.));
#4672=DIRECTION('center_axis',(0.,1.,0.));
#4673=DIRECTION('ref_axis',(1.,0.,0.));
#4674=DIRECTION('center_axis',(0.,-1.,0.));
#4675=DIRECTION('ref_axis',(1.,0.,0.));
#4676=DIRECTION('center_axis',(0.,-1.,0.));
#4677=DIRECTION('ref_axis',(0.,0.,-1.));
#4678=DIRECTION('center_axis',(0.,0.,1.));
#4679=DIRECTION('ref_axis',(1.,0.,0.));
#4680=DIRECTION('center_axis',(0.,-1.,0.));
#4681=DIRECTION('ref_axis',(0.,0.,-1.));
#4682=DIRECTION('center_axis',(0.,1.,0.));
#4683=DIRECTION('ref_axis',(1.,0.,0.));
#4684=DIRECTION('center_axis',(0.,-1.,0.));
#4685=DIRECTION('ref_axis',(1.,0.,0.));
#4686=DIRECTION('center_axis',(0.,-1.,0.));
#4687=DIRECTION('ref_axis',(0.,0.,-1.));
#4688=DIRECTION('center_axis',(0.,0.,1.));
#4689=DIRECTION('ref_axis',(1.,0.,0.));
#4690=DIRECTION('center_axis',(0.,-1.,0.));
#4691=DIRECTION('ref_axis',(0.,0.,-1.));
#4692=DIRECTION('center_axis',(0.,1.,0.));
#4693=DIRECTION('ref_axis',(1.,0.,0.));
#4694=DIRECTION('center_axis',(0.,-1.,0.));
#4695=DIRECTION('ref_axis',(1.,0.,0.));
#4696=DIRECTION('center_axis',(0.,-1.,0.));
#4697=DIRECTION('ref_axis',(0.,0.,-1.));
#4698=DIRECTION('center_axis',(6.12323399573676E-17,0.,1.));
#4699=DIRECTION('ref_axis',(1.,0.,0.));
#4700=DIRECTION('center_axis',(0.,-1.,0.));
#4701=DIRECTION('ref_axis',(0.,0.,-1.));
#4702=DIRECTION('center_axis',(0.,1.,0.));
#4703=DIRECTION('ref_axis',(1.,0.,0.));
#4704=DIRECTION('center_axis',(0.,-1.,0.));
#4705=DIRECTION('ref_axis',(1.,0.,0.));
#4706=DIRECTION('center_axis',(0.,-1.,0.));
#4707=DIRECTION('ref_axis',(0.,0.,-1.));
#4708=DIRECTION('center_axis',(0.,0.,1.));
#4709=DIRECTION('ref_axis',(1.,0.,0.));
#4710=DIRECTION('center_axis',(0.,-1.,0.));
#4711=DIRECTION('ref_axis',(0.,0.,-1.));
#4712=DIRECTION('center_axis',(0.,1.,0.));
#4713=DIRECTION('ref_axis',(1.,0.,0.));
#4714=DIRECTION('center_axis',(0.,1.,0.));
#4715=DIRECTION('ref_axis',(1.,0.,0.));
#4716=DIRECTION('',(0.,1.,0.));
#4717=DIRECTION('center_axis',(0.,-1.,0.));
#4718=DIRECTION('ref_axis',(1.,0.,0.));
#4719=DIRECTION('center_axis',(0.,-1.,0.));
#4720=DIRECTION('ref_axis',(1.,0.,0.));
#4721=DIRECTION('center_axis',(0.,1.,0.));
#4722=DIRECTION('ref_axis',(1.,0.,0.));
#4723=DIRECTION('center_axis',(0.,-1.,0.));
#4724=DIRECTION('ref_axis',(0.,0.,-1.));
#4725=DIRECTION('center_axis',(0.,0.,1.));
#4726=DIRECTION('ref_axis',(1.,0.,0.));
#4727=DIRECTION('center_axis',(0.,-1.,0.));
#4728=DIRECTION('ref_axis',(0.,0.,-1.));
#4729=DIRECTION('center_axis',(0.,-1.,0.));
#4730=DIRECTION('ref_axis',(-1.,0.,0.));
#4731=DIRECTION('center_axis',(0.,1.,0.));
#4732=DIRECTION('ref_axis',(1.,0.,0.));
#5769=CARTESIAN_POINT('',(0.,0.,0.));
#5770=CARTESIAN_POINT('Origin',(0.707106781186547,0.,0.707106781186548));
#5771=CARTESIAN_POINT('',(0.504455939115715,-0.04763,0.841298510752802));
#5772=CARTESIAN_POINT('',(0.841298510752802,-0.04763,0.504455939115715));
#5773=CARTESIAN_POINT('Ctrl Pts',(0.504455939115715,-0.04763,0.841298510752802));
#5774=CARTESIAN_POINT('Ctrl Pts',(0.508899795931835,-0.0740444353928835,
0.838633903678357));
#5775=CARTESIAN_POINT('Ctrl Pts',(0.517157748491652,-0.0999305678883309,
0.833661031856294));
#5776=CARTESIAN_POINT('Ctrl Pts',(0.537715343527944,-0.142345102874864,
0.820511285096538));
#5777=CARTESIAN_POINT('Ctrl Pts',(0.548874290046456,-0.159766064500479,
0.813159949759));
#5778=CARTESIAN_POINT('Ctrl Pts',(0.573915184558107,-0.190326085855194,
0.795684265985089));
#5779=CARTESIAN_POINT('Ctrl Pts',(0.587792702767295,-0.203463743702801,
0.78555112003688));
#5780=CARTESIAN_POINT('Ctrl Pts',(0.615966552324775,-0.224161999508995,
0.763642258217233));
#5781=CARTESIAN_POINT('Ctrl Pts',(0.631684198665438,-0.232861760990032,
0.750785745543687));
#5782=CARTESIAN_POINT('Ctrl Pts',(0.663382628119203,-0.244251601209411,
0.722929908501543));
#5783=CARTESIAN_POINT('Ctrl Pts',(0.679352081686668,-0.246942143572133,
0.707917883896095));
#5784=CARTESIAN_POINT('Ctrl Pts',(0.707917883896095,-0.246942143572133,
0.679352081686668));
#5785=CARTESIAN_POINT('Ctrl Pts',(0.722929908501543,-0.244251601209411,
0.663382628119203));
#5786=CARTESIAN_POINT('Ctrl Pts',(0.750785745543687,-0.232861760990032,
0.631684198665439));
#5787=CARTESIAN_POINT('Ctrl Pts',(0.763642258217232,-0.224161999508995,
0.615966552324775));
#5788=CARTESIAN_POINT('Ctrl Pts',(0.78555112003688,-0.203463743702801,0.587792702767295));
#5789=CARTESIAN_POINT('Ctrl Pts',(0.795684265985088,-0.190326085855194,
0.573915184558108));
#5790=CARTESIAN_POINT('Ctrl Pts',(0.813159949759,-0.15976606450048,0.548874290046456));
#5791=CARTESIAN_POINT('Ctrl Pts',(0.820511285096538,-0.142345102874864,
0.537715343527944));
#5792=CARTESIAN_POINT('Ctrl Pts',(0.833661031856294,-0.099930567888331,
0.517157748491653));
#5793=CARTESIAN_POINT('Ctrl Pts',(0.838633903678357,-0.0740444353928835,
0.508899795931835));
#5794=CARTESIAN_POINT('Ctrl Pts',(0.841298510752801,-0.0476299999999999,
0.504455939115715));
#5795=CARTESIAN_POINT('',(0.528110872004958,-0.04763,0.871530771444223));
#5796=CARTESIAN_POINT('Origin',(0.707106781186547,-0.04763,0.707106781186548));
#5797=CARTESIAN_POINT('',(0.871530771444223,-0.04763,0.528110872004959));
#5798=CARTESIAN_POINT('Ctrl Pts',(0.871530771444223,-0.0476300000000001,
0.528110872004958));
#5799=CARTESIAN_POINT('Ctrl Pts',(0.87014664509073,-0.0609922781173483,
0.530395067942936));
#5800=CARTESIAN_POINT('Ctrl Pts',(0.868149331745851,-0.0742967091364493,
0.533674141594226));
#5801=CARTESIAN_POINT('Ctrl Pts',(0.85981294420286,-0.115492077056649,0.54708917182331));
#5802=CARTESIAN_POINT('Ctrl Pts',(0.850993704737257,-0.141695629206859,
0.560922177770136));
#5803=CARTESIAN_POINT('Ctrl Pts',(0.830754510485543,-0.181890537957859,
0.590422647829571));
#5804=CARTESIAN_POINT('Ctrl Pts',(0.816896541396381,-0.201072148666545,
0.609616703125488));
#5805=CARTESIAN_POINT('Ctrl Pts',(0.792310597819928,-0.223955109275652,
0.641117951819998));
#5806=CARTESIAN_POINT('Ctrl Pts',(0.779109323683612,-0.232742381310829,
0.657208095763053));
#5807=CARTESIAN_POINT('Ctrl Pts',(0.750552691816206,-0.244234834628584,
0.68964083160521));
#5808=CARTESIAN_POINT('Ctrl Pts',(0.735185187071673,-0.246942143572133,
0.705971972091755));
#5809=CARTESIAN_POINT('Ctrl Pts',(0.705971972091754,-0.246942143572133,
0.735185187071673));
#5810=CARTESIAN_POINT('Ctrl Pts',(0.689640831605209,-0.244234834628584,
0.750552691816206));
#5811=CARTESIAN_POINT('Ctrl Pts',(0.657208095763052,-0.232742381310829,
0.779109323683612));
#5812=CARTESIAN_POINT('Ctrl Pts',(0.641117951819998,-0.223955109275652,
0.792310597819928));
#5813=CARTESIAN_POINT('Ctrl Pts',(0.609616703125487,-0.201072148666545,
0.816896541396382));
#5814=CARTESIAN_POINT('Ctrl Pts',(0.590422647829571,-0.181890537957858,
0.830754510485544));
#5815=CARTESIAN_POINT('Ctrl Pts',(0.560922177770135,-0.141695629206858,
0.850993704737257));
#5816=CARTESIAN_POINT('Ctrl Pts',(0.547089171823309,-0.115492077056649,
0.859812944202861));
#5817=CARTESIAN_POINT('Ctrl Pts',(0.533674141594226,-0.0742967091364491,
0.868149331745852));
#5818=CARTESIAN_POINT('Ctrl Pts',(0.530395067942936,-0.0609922781173483,
0.870146645090731));
#5819=CARTESIAN_POINT('Ctrl Pts',(0.528110872004958,-0.0476300000000001,
0.871530771444223));
#5820=CARTESIAN_POINT('Origin',(0.707106781186547,-0.04763,0.707106781186548));
#5821=CARTESIAN_POINT('Origin',(0.,-0.166705,0.));
#5822=CARTESIAN_POINT('',(0.242834539687906,-0.04763,0.989696097314));
#5823=CARTESIAN_POINT('Origin',(0.,-0.04763,0.));
#5824=CARTESIAN_POINT('',(-0.242834539687907,-0.04763,0.989696097314));
#5825=CARTESIAN_POINT('Ctrl Pts',(0.242834539687906,-0.04763,0.989696097314));
#5826=CARTESIAN_POINT('Ctrl Pts',(0.24024064412003,-0.0609922781173483,
0.990332542620729));
#5827=CARTESIAN_POINT('Ctrl Pts',(0.236509675094874,-0.0742967091364492,
0.991238884025248));
#5828=CARTESIAN_POINT('Ctrl Pts',(0.221129100087819,-0.115492077056649,
0.994830026707808));
#5829=CARTESIAN_POINT('Ctrl Pts',(0.205111543747588,-0.141695629206859,
0.998375294985966));
#5830=CARTESIAN_POINT('Ctrl Pts',(0.169940289819232,-0.181890537957859,
1.00492400591205));
#5831=CARTESIAN_POINT('Ctrl Pts',(0.1465689792446,-0.201072148666545,1.00869718865384));
#5832=CARTESIAN_POINT('Ctrl Pts',(0.106909345252087,-0.223955109275652,
1.01358704779679));
#5833=CARTESIAN_POINT('Ctrl Pts',(0.0861971848975941,-0.232742381310829,
1.0156297872271));
#5834=CARTESIAN_POINT('Ctrl Pts',(0.0430711894098822,-0.244234834628584,
1.01837060663223));
#5835=CARTESIAN_POINT('Ctrl Pts',(0.0206568624125605,-0.246942143572133,
1.019052));
#5836=CARTESIAN_POINT('Ctrl Pts',(-0.0206568624125608,-0.246942143572133,
1.019052));
#5837=CARTESIAN_POINT('Ctrl Pts',(-0.0430711894098825,-0.244234834628584,
1.01837060663223));
#5838=CARTESIAN_POINT('Ctrl Pts',(-0.0861971848975943,-0.232742381310829,
1.0156297872271));
#5839=CARTESIAN_POINT('Ctrl Pts',(-0.106909345252088,-0.223955109275652,
1.01358704779679));
#5840=CARTESIAN_POINT('Ctrl Pts',(-0.1465689792446,-0.201072148666545,1.00869718865384));
#5841=CARTESIAN_POINT('Ctrl Pts',(-0.169940289819232,-0.181890537957859,
1.00492400591205));
#5842=CARTESIAN_POINT('Ctrl Pts',(-0.205111543747588,-0.141695629206859,
0.998375294985966));
#5843=CARTESIAN_POINT('Ctrl Pts',(-0.221129100087819,-0.115492077056649,
0.994830026707808));
#5844=CARTESIAN_POINT('Ctrl Pts',(-0.236509675094875,-0.0742967091364493,
0.991238884025248));
#5845=CARTESIAN_POINT('Ctrl Pts',(-0.24024064412003,-0.0609922781173483,
0.990332542620729));
#5846=CARTESIAN_POINT('Ctrl Pts',(-0.242834539687907,-0.04763,0.989696097314));
#5847=CARTESIAN_POINT('',(-0.528110872004959,-0.04763,0.871530771444223));
#5848=CARTESIAN_POINT('Origin',(0.,-0.04763,0.));
#5849=CARTESIAN_POINT('',(-0.871530771444223,-0.04763,0.528110872004958));
#5850=CARTESIAN_POINT('Ctrl Pts',(-0.528110872004958,-0.0476300000000001,
0.871530771444223));
#5851=CARTESIAN_POINT('Ctrl Pts',(-0.530395067942936,-0.0609922781173484,
0.87014664509073));
#5852=CARTESIAN_POINT('Ctrl Pts',(-0.533674141594226,-0.0742967091364493,
0.868149331745851));
#5853=CARTESIAN_POINT('Ctrl Pts',(-0.54708917182331,-0.115492077056649,
0.85981294420286));
#5854=CARTESIAN_POINT('Ctrl Pts',(-0.560922177770136,-0.141695629206859,
0.850993704737257));
#5855=CARTESIAN_POINT('Ctrl Pts',(-0.590422647829571,-0.181890537957859,
0.830754510485543));
#5856=CARTESIAN_POINT('Ctrl Pts',(-0.609616703125488,-0.201072148666545,
0.816896541396381));
#5857=CARTESIAN_POINT('Ctrl Pts',(-0.641117951819998,-0.223955109275652,
0.792310597819928));
#5858=CARTESIAN_POINT('Ctrl Pts',(-0.657208095763053,-0.232742381310829,
0.779109323683611));
#5859=CARTESIAN_POINT('Ctrl Pts',(-0.68964083160521,-0.244234834628584,
0.750552691816205));
#5860=CARTESIAN_POINT('Ctrl Pts',(-0.705971972091755,-0.246942143572133,
0.735185187071673));
#5861=CARTESIAN_POINT('Ctrl Pts',(-0.735185187071673,-0.246942143572133,
0.705971972091754));
#5862=CARTESIAN_POINT('Ctrl Pts',(-0.750552691816206,-0.244234834628584,
0.689640831605209));
#5863=CARTESIAN_POINT('Ctrl Pts',(-0.779109323683612,-0.232742381310829,
0.657208095763052));
#5864=CARTESIAN_POINT('Ctrl Pts',(-0.792310597819928,-0.223955109275652,
0.641117951819998));
#5865=CARTESIAN_POINT('Ctrl Pts',(-0.816896541396382,-0.201072148666545,
0.609616703125487));
#5866=CARTESIAN_POINT('Ctrl Pts',(-0.830754510485544,-0.181890537957858,
0.590422647829571));
#5867=CARTESIAN_POINT('Ctrl Pts',(-0.850993704737257,-0.141695629206858,
0.560922177770135));
#5868=CARTESIAN_POINT('Ctrl Pts',(-0.859812944202861,-0.115492077056649,
0.547089171823309));
#5869=CARTESIAN_POINT('Ctrl Pts',(-0.868149331745852,-0.0742967091364491,
0.533674141594226));
#5870=CARTESIAN_POINT('Ctrl Pts',(-0.870146645090731,-0.0609922781173483,
0.530395067942936));
#5871=CARTESIAN_POINT('Ctrl Pts',(-0.871530771444223,-0.04763,0.528110872004958));
#5872=CARTESIAN_POINT('',(-0.989696097314,-0.04763,0.242834539687906));
#5873=CARTESIAN_POINT('Origin',(0.,-0.04763,0.));
#5874=CARTESIAN_POINT('',(-1.019052,-0.246942143572133,1.248489836334E-16));
#5875=CARTESIAN_POINT('Ctrl Pts',(-0.989696097314,-0.04763,0.242834539687906));
#5876=CARTESIAN_POINT('Ctrl Pts',(-0.990332542620729,-0.0609922781173483,
0.24024064412003));
#5877=CARTESIAN_POINT('Ctrl Pts',(-0.991238884025248,-0.0742967091364492,
0.236509675094874));
#5878=CARTESIAN_POINT('Ctrl Pts',(-0.994830026707808,-0.115492077056649,
0.221129100087819));
#5879=CARTESIAN_POINT('Ctrl Pts',(-0.998375294985966,-0.141695629206859,
0.205111543747588));
#5880=CARTESIAN_POINT('Ctrl Pts',(-1.00492400591205,-0.181890537957859,
0.169940289819232));
#5881=CARTESIAN_POINT('Ctrl Pts',(-1.00869718865384,-0.201072148666545,
0.1465689792446));
#5882=CARTESIAN_POINT('Ctrl Pts',(-1.01358704779679,-0.223955109275652,
0.106909345252088));
#5883=CARTESIAN_POINT('Ctrl Pts',(-1.0156297872271,-0.232742381310829,0.0861971848975944));
#5884=CARTESIAN_POINT('Ctrl Pts',(-1.01837060663223,-0.244234834628584,
0.0430711894098825));
#5885=CARTESIAN_POINT('Ctrl Pts',(-1.019052,-0.246942143572133,0.0206568624125608));
#5886=CARTESIAN_POINT('Ctrl Pts',(-1.019052,-0.246942143572133,1.2490009027033E-16));
#5887=CARTESIAN_POINT('',(-1.019052,-0.28578,1.24797876996471E-16));
#5888=CARTESIAN_POINT('',(-1.019052,-0.166705,1.24797876996471E-16));
#5889=CARTESIAN_POINT('Origin',(0.,-0.28578,0.));
#5890=CARTESIAN_POINT('',(-0.989696097314,-0.04763,-0.242834539687906));
#5891=CARTESIAN_POINT('Ctrl Pts',(-1.019052,-0.246942143572133,1.2490009027033E-16));
#5892=CARTESIAN_POINT('Ctrl Pts',(-1.019052,-0.246942143572133,-0.0206568624125605));
#5893=CARTESIAN_POINT('Ctrl Pts',(-1.01837060663223,-0.244234834628584,
-0.0430711894098822));
#5894=CARTESIAN_POINT('Ctrl Pts',(-1.0156297872271,-0.232742381310829,-0.0861971848975941));
#5895=CARTESIAN_POINT('Ctrl Pts',(-1.01358704779679,-0.223955109275652,
-0.106909345252087));
#5896=CARTESIAN_POINT('Ctrl Pts',(-1.00869718865384,-0.201072148666546,
-0.1465689792446));
#5897=CARTESIAN_POINT('Ctrl Pts',(-1.00492400591205,-0.181890537957859,
-0.169940289819232));
#5898=CARTESIAN_POINT('Ctrl Pts',(-0.998375294985966,-0.141695629206859,
-0.205111543747588));
#5899=CARTESIAN_POINT('Ctrl Pts',(-0.994830026707808,-0.11549207705665,
-0.221129100087819));
#5900=CARTESIAN_POINT('Ctrl Pts',(-0.991238884025248,-0.0742967091364495,
-0.236509675094874));
#5901=CARTESIAN_POINT('Ctrl Pts',(-0.990332542620729,-0.0609922781173484,
-0.24024064412003));
#5902=CARTESIAN_POINT('Ctrl Pts',(-0.989696097314,-0.0476300000000001,-0.242834539687907));
#5903=CARTESIAN_POINT('',(-0.871530771444223,-0.04763,-0.528110872004958));
#5904=CARTESIAN_POINT('Origin',(0.,-0.04763,0.));
#5905=CARTESIAN_POINT('',(-0.528110872004958,-0.04763,-0.871530771444223));
#5906=CARTESIAN_POINT('Ctrl Pts',(-0.871530771444223,-0.0476300000000001,
-0.528110872004958));
#5907=CARTESIAN_POINT('Ctrl Pts',(-0.87014664509073,-0.0609922781173484,
-0.530395067942936));
#5908=CARTESIAN_POINT('Ctrl Pts',(-0.868149331745851,-0.0742967091364494,
-0.533674141594226));
#5909=CARTESIAN_POINT('Ctrl Pts',(-0.85981294420286,-0.115492077056649,
-0.54708917182331));
#5910=CARTESIAN_POINT('Ctrl Pts',(-0.850993704737257,-0.141695629206859,
-0.560922177770136));
#5911=CARTESIAN_POINT('Ctrl Pts',(-0.830754510485543,-0.181890537957859,
-0.590422647829571));
#5912=CARTESIAN_POINT('Ctrl Pts',(-0.816896541396381,-0.201072148666546,
-0.609616703125488));
#5913=CARTESIAN_POINT('Ctrl Pts',(-0.792310597819928,-0.223955109275652,
-0.641117951819999));
#5914=CARTESIAN_POINT('Ctrl Pts',(-0.779109323683611,-0.232742381310829,
-0.657208095763053));
#5915=CARTESIAN_POINT('Ctrl Pts',(-0.750552691816205,-0.244234834628584,
-0.68964083160521));
#5916=CARTESIAN_POINT('Ctrl Pts',(-0.735185187071673,-0.246942143572133,
-0.705971972091755));
#5917=CARTESIAN_POINT('Ctrl Pts',(-0.705971972091754,-0.246942143572133,
-0.735185187071673));
#5918=CARTESIAN_POINT('Ctrl Pts',(-0.68964083160521,-0.244234834628584,
-0.750552691816206));
#5919=CARTESIAN_POINT('Ctrl Pts',(-0.657208095763052,-0.232742381310829,
-0.779109323683612));
#5920=CARTESIAN_POINT('Ctrl Pts',(-0.641117951819998,-0.223955109275652,
-0.792310597819928));
#5921=CARTESIAN_POINT('Ctrl Pts',(-0.609616703125488,-0.201072148666545,
-0.816896541396381));
#5922=CARTESIAN_POINT('Ctrl Pts',(-0.590422647829571,-0.181890537957859,
-0.830754510485543));
#5923=CARTESIAN_POINT('Ctrl Pts',(-0.560922177770136,-0.141695629206859,
-0.850993704737257));
#5924=CARTESIAN_POINT('Ctrl Pts',(-0.54708917182331,-0.115492077056649,
-0.85981294420286));
#5925=CARTESIAN_POINT('Ctrl Pts',(-0.533674141594226,-0.0742967091364494,
-0.868149331745852));
#5926=CARTESIAN_POINT('Ctrl Pts',(-0.530395067942936,-0.0609922781173484,
-0.870146645090731));
#5927=CARTESIAN_POINT('Ctrl Pts',(-0.528110872004958,-0.0476300000000001,
-0.871530771444223));
#5928=CARTESIAN_POINT('',(-0.242834539687906,-0.04763,-0.989696097314));
#5929=CARTESIAN_POINT('Origin',(0.,-0.04763,0.));
#5930=CARTESIAN_POINT('',(0.242834539687906,-0.04763,-0.989696097314));
#5931=CARTESIAN_POINT('Ctrl Pts',(-0.242834539687907,-0.04763,-0.989696097314));
#5932=CARTESIAN_POINT('Ctrl Pts',(-0.24024064412003,-0.0609922781173483,
-0.990332542620729));
#5933=CARTESIAN_POINT('Ctrl Pts',(-0.236509675094874,-0.0742967091364493,
-0.991238884025248));
#5934=CARTESIAN_POINT('Ctrl Pts',(-0.221129100087819,-0.115492077056649,
-0.994830026707808));
#5935=CARTESIAN_POINT('Ctrl Pts',(-0.205111543747588,-0.141695629206859,
-0.998375294985966));
#5936=CARTESIAN_POINT('Ctrl Pts',(-0.169940289819232,-0.181890537957859,
-1.00492400591205));
#5937=CARTESIAN_POINT('Ctrl Pts',(-0.1465689792446,-0.201072148666545,-1.00869718865384));
#5938=CARTESIAN_POINT('Ctrl Pts',(-0.106909345252087,-0.223955109275652,
-1.01358704779679));
#5939=CARTESIAN_POINT('Ctrl Pts',(-0.0861971848975942,-0.232742381310829,
-1.0156297872271));
#5940=CARTESIAN_POINT('Ctrl Pts',(-0.0430711894098823,-0.244234834628584,
-1.01837060663223));
#5941=CARTESIAN_POINT('Ctrl Pts',(-0.0206568624125606,-0.246942143572133,
-1.019052));
#5942=CARTESIAN_POINT('Ctrl Pts',(0.0206568624125607,-0.246942143572133,
-1.019052));
#5943=CARTESIAN_POINT('Ctrl Pts',(0.0430711894098824,-0.244234834628584,
-1.01837060663223));
#5944=CARTESIAN_POINT('Ctrl Pts',(0.0861971848975943,-0.232742381310829,
-1.0156297872271));
#5945=CARTESIAN_POINT('Ctrl Pts',(0.106909345252088,-0.223955109275652,
-1.01358704779679));
#5946=CARTESIAN_POINT('Ctrl Pts',(0.1465689792446,-0.201072148666545,-1.00869718865384));
#5947=CARTESIAN_POINT('Ctrl Pts',(0.169940289819232,-0.181890537957859,
-1.00492400591205));
#5948=CARTESIAN_POINT('Ctrl Pts',(0.205111543747588,-0.141695629206859,
-0.998375294985966));
#5949=CARTESIAN_POINT('Ctrl Pts',(0.221129100087819,-0.115492077056649,
-0.994830026707808));
#5950=CARTESIAN_POINT('Ctrl Pts',(0.236509675094874,-0.0742967091364493,
-0.991238884025248));
#5951=CARTESIAN_POINT('Ctrl Pts',(0.24024064412003,-0.0609922781173484,
-0.990332542620729));
#5952=CARTESIAN_POINT('Ctrl Pts',(0.242834539687907,-0.04763,-0.989696097314));
#5953=CARTESIAN_POINT('',(0.528110872004958,-0.04763,-0.871530771444223));
#5954=CARTESIAN_POINT('Origin',(0.,-0.04763,0.));
#5955=CARTESIAN_POINT('',(0.871530771444223,-0.04763,-0.528110872004958));
#5956=CARTESIAN_POINT('Ctrl Pts',(0.528110872004958,-0.0476300000000001,
-0.871530771444223));
#5957=CARTESIAN_POINT('Ctrl Pts',(0.530395067942936,-0.0609922781173484,
-0.870146645090731));
#5958=CARTESIAN_POINT('Ctrl Pts',(0.533674141594226,-0.0742967091364493,
-0.868149331745851));
#5959=CARTESIAN_POINT('Ctrl Pts',(0.54708917182331,-0.115492077056649,-0.85981294420286));
#5960=CARTESIAN_POINT('Ctrl Pts',(0.560922177770136,-0.141695629206859,
-0.850993704737257));
#5961=CARTESIAN_POINT('Ctrl Pts',(0.590422647829571,-0.181890537957859,
-0.830754510485543));
#5962=CARTESIAN_POINT('Ctrl Pts',(0.609616703125488,-0.201072148666545,
-0.816896541396381));
#5963=CARTESIAN_POINT('Ctrl Pts',(0.641117951819998,-0.223955109275652,
-0.792310597819928));
#5964=CARTESIAN_POINT('Ctrl Pts',(0.657208095763053,-0.232742381310829,
-0.779109323683612));
#5965=CARTESIAN_POINT('Ctrl Pts',(0.68964083160521,-0.244234834628584,-0.750552691816206));
#5966=CARTESIAN_POINT('Ctrl Pts',(0.705971972091755,-0.246942143572133,
-0.735185187071673));
#5967=CARTESIAN_POINT('Ctrl Pts',(0.735185187071673,-0.246942143572133,
-0.705971972091754));
#5968=CARTESIAN_POINT('Ctrl Pts',(0.750552691816206,-0.244234834628584,
-0.68964083160521));
#5969=CARTESIAN_POINT('Ctrl Pts',(0.779109323683612,-0.232742381310829,
-0.657208095763053));
#5970=CARTESIAN_POINT('Ctrl Pts',(0.792310597819928,-0.223955109275652,
-0.641117951819998));
#5971=CARTESIAN_POINT('Ctrl Pts',(0.816896541396381,-0.201072148666545,
-0.609616703125488));
#5972=CARTESIAN_POINT('Ctrl Pts',(0.830754510485543,-0.181890537957859,
-0.590422647829571));
#5973=CARTESIAN_POINT('Ctrl Pts',(0.850993704737257,-0.141695629206859,
-0.560922177770136));
#5974=CARTESIAN_POINT('Ctrl Pts',(0.85981294420286,-0.115492077056649,-0.54708917182331));
#5975=CARTESIAN_POINT('Ctrl Pts',(0.868149331745851,-0.0742967091364493,
-0.533674141594226));
#5976=CARTESIAN_POINT('Ctrl Pts',(0.870146645090731,-0.0609922781173484,
-0.530395067942936));
#5977=CARTESIAN_POINT('Ctrl Pts',(0.871530771444223,-0.0476300000000001,
-0.528110872004958));
#5978=CARTESIAN_POINT('',(0.989696097314,-0.04763,-0.242834539687906));
#5979=CARTESIAN_POINT('Origin',(0.,-0.04763,0.));
#5980=CARTESIAN_POINT('',(0.989696097314,-0.04763,0.242834539687906));
#5981=CARTESIAN_POINT('Ctrl Pts',(0.989696097314,-0.04763,-0.242834539687907));
#5982=CARTESIAN_POINT('Ctrl Pts',(0.990332542620729,-0.0609922781173483,
-0.24024064412003));
#5983=CARTESIAN_POINT('Ctrl Pts',(0.991238884025248,-0.0742967091364493,
-0.236509675094874));
#5984=CARTESIAN_POINT('Ctrl Pts',(0.994830026707808,-0.115492077056649,
-0.221129100087819));
#5985=CARTESIAN_POINT('Ctrl Pts',(0.998375294985966,-0.141695629206859,
-0.205111543747588));
#5986=CARTESIAN_POINT('Ctrl Pts',(1.00492400591205,-0.181890537957859,-0.169940289819232));
#5987=CARTESIAN_POINT('Ctrl Pts',(1.00869718865384,-0.201072148666545,-0.1465689792446));
#5988=CARTESIAN_POINT('Ctrl Pts',(1.01358704779679,-0.223955109275652,-0.106909345252087));
#5989=CARTESIAN_POINT('Ctrl Pts',(1.0156297872271,-0.232742381310829,-0.0861971848975942));
#5990=CARTESIAN_POINT('Ctrl Pts',(1.01837060663223,-0.244234834628584,-0.0430711894098823));
#5991=CARTESIAN_POINT('Ctrl Pts',(1.019052,-0.246942143572133,-0.0206568624125607));
#5992=CARTESIAN_POINT('Ctrl Pts',(1.019052,-0.246942143572133,0.0206568624125607));
#5993=CARTESIAN_POINT('Ctrl Pts',(1.01837060663223,-0.244234834628584,0.0430711894098823));
#5994=CARTESIAN_POINT('Ctrl Pts',(1.0156297872271,-0.232742381310829,0.0861971848975942));
#5995=CARTESIAN_POINT('Ctrl Pts',(1.01358704779679,-0.223955109275652,0.106909345252087));
#5996=CARTESIAN_POINT('Ctrl Pts',(1.00869718865384,-0.201072148666545,0.1465689792446));
#5997=CARTESIAN_POINT('Ctrl Pts',(1.00492400591205,-0.181890537957859,0.169940289819232));
#5998=CARTESIAN_POINT('Ctrl Pts',(0.998375294985966,-0.141695629206859,
0.205111543747588));
#5999=CARTESIAN_POINT('Ctrl Pts',(0.994830026707808,-0.115492077056649,
0.221129100087819));
#6000=CARTESIAN_POINT('Ctrl Pts',(0.991238884025248,-0.0742967091364492,
0.236509675094874));
#6001=CARTESIAN_POINT('Ctrl Pts',(0.990332542620729,-0.0609922781173483,
0.24024064412003));
#6002=CARTESIAN_POINT('Ctrl Pts',(0.989696097314,-0.04763,0.242834539687907));
#6003=CARTESIAN_POINT('Origin',(0.,-0.04763,0.));
#6004=CARTESIAN_POINT('Origin',(0.,-0.04763,0.));
#6005=CARTESIAN_POINT('',(0.238183666596899,-0.04763,0.951592097314));
#6006=CARTESIAN_POINT('Origin',(0.,-0.04763,0.));
#6007=CARTESIAN_POINT('Origin',(-1.94289029309402E-16,-0.04763,1.));
#6008=CARTESIAN_POINT('Origin',(-1.94289029309402E-16,0.,1.));
#6009=CARTESIAN_POINT('',(-0.2381836665969,-0.04763,0.951592097314));
#6010=CARTESIAN_POINT('Ctrl Pts',(-0.238183666596899,-0.0476299999999999,
0.951592097314));
#6011=CARTESIAN_POINT('Ctrl Pts',(-0.233157223576062,-0.0740444353928835,
0.952850216871763));
#6012=CARTESIAN_POINT('Ctrl Pts',(-0.223801617934946,-0.0999305678883309,
0.955173119738174));
#6013=CARTESIAN_POINT('Ctrl Pts',(-0.199966927975188,-0.142345102874864,
0.960411259488514));
#6014=CARTESIAN_POINT('Ctrl Pts',(-0.1868781821531,-0.159766064500479,0.963103647174702));
#6015=CARTESIAN_POINT('Ctrl Pts',(-0.15681442133453,-0.190326085855194,
0.968453058988463));
#6016=CARTESIAN_POINT('Ctrl Pts',(-0.139836317888043,-0.203463743702801,
0.971100730005489));
#6017=CARTESIAN_POINT('Ctrl Pts',(-0.104422493053067,-0.224161999508995,
0.975530745318961));
#6018=CARTESIAN_POINT('Ctrl Pts',(-0.0842175114474176,-0.232861760990032,
0.977553872336861));
#6019=CARTESIAN_POINT('Ctrl Pts',(-0.0421062857595701,-0.244251601209411,
0.980270995488453));
#6020=CARTESIAN_POINT('Ctrl Pts',(-0.0201990724523197,-0.246942143572133,
0.980948));
#6021=CARTESIAN_POINT('Ctrl Pts',(0.020199072452319,-0.246942143572133,
0.980948));
#6022=CARTESIAN_POINT('Ctrl Pts',(0.0421062857595694,-0.244251601209411,
0.980270995488454));
#6023=CARTESIAN_POINT('Ctrl Pts',(0.0842175114474169,-0.232861760990032,
0.977553872336861));
#6024=CARTESIAN_POINT('Ctrl Pts',(0.104422493053067,-0.224161999508995,
0.975530745318961));
#6025=CARTESIAN_POINT('Ctrl Pts',(0.139836317888042,-0.203463743702801,
0.971100730005489));
#6026=CARTESIAN_POINT('Ctrl Pts',(0.15681442133453,-0.190326085855194,0.968453058988463));
#6027=CARTESIAN_POINT('Ctrl Pts',(0.1868781821531,-0.15976606450048,0.963103647174702));
#6028=CARTESIAN_POINT('Ctrl Pts',(0.199966927975188,-0.142345102874864,
0.960411259488514));
#6029=CARTESIAN_POINT('Ctrl Pts',(0.223801617934945,-0.0999305678883309,
0.955173119738174));
#6030=CARTESIAN_POINT('Ctrl Pts',(0.233157223576061,-0.0740444353928835,
0.952850216871763));
#6031=CARTESIAN_POINT('Ctrl Pts',(0.238183666596899,-0.0476299999999999,
0.951592097314));
#6032=CARTESIAN_POINT('Origin',(-1.94289029309402E-16,-0.04763,1.));
#6033=CARTESIAN_POINT('Origin',(0.,-0.04763,0.));
#6034=CARTESIAN_POINT('',(-0.504455939115715,-0.04763,0.841298510752802));
#6035=CARTESIAN_POINT('Origin',(0.,-0.04763,0.));
#6036=CARTESIAN_POINT('Origin',(-0.707106781186548,-0.04763,0.707106781186547));
#6037=CARTESIAN_POINT('Origin',(-0.707106781186548,0.,0.707106781186547));
#6038=CARTESIAN_POINT('',(-0.841298510752802,-0.04763,0.504455939115715));
#6039=CARTESIAN_POINT('Ctrl Pts',(-0.841298510752802,-0.04763,0.504455939115715));
#6040=CARTESIAN_POINT('Ctrl Pts',(-0.838633903678357,-0.0740444353928835,
0.508899795931835));
#6041=CARTESIAN_POINT('Ctrl Pts',(-0.833661031856294,-0.0999305678883309,
0.517157748491652));
#6042=CARTESIAN_POINT('Ctrl Pts',(-0.820511285096538,-0.142345102874864,
0.537715343527944));
#6043=CARTESIAN_POINT('Ctrl Pts',(-0.813159949759,-0.159766064500479,0.548874290046456));
#6044=CARTESIAN_POINT('Ctrl Pts',(-0.795684265985089,-0.190326085855194,
0.573915184558107));
#6045=CARTESIAN_POINT('Ctrl Pts',(-0.78555112003688,-0.203463743702801,
0.587792702767295));
#6046=CARTESIAN_POINT('Ctrl Pts',(-0.763642258217233,-0.224161999508995,
0.615966552324775));
#6047=CARTESIAN_POINT('Ctrl Pts',(-0.750785745543687,-0.232861760990032,
0.631684198665438));
#6048=CARTESIAN_POINT('Ctrl Pts',(-0.722929908501543,-0.244251601209411,
0.663382628119203));
#6049=CARTESIAN_POINT('Ctrl Pts',(-0.707917883896095,-0.246942143572133,
0.679352081686668));
#6050=CARTESIAN_POINT('Ctrl Pts',(-0.679352081686668,-0.246942143572133,
0.707917883896095));
#6051=CARTESIAN_POINT('Ctrl Pts',(-0.663382628119203,-0.244251601209411,
0.722929908501544));
#6052=CARTESIAN_POINT('Ctrl Pts',(-0.631684198665438,-0.232861760990031,
0.750785745543687));
#6053=CARTESIAN_POINT('Ctrl Pts',(-0.615966552324775,-0.224161999508995,
0.763642258217233));
#6054=CARTESIAN_POINT('Ctrl Pts',(-0.587792702767295,-0.203463743702801,
0.78555112003688));
#6055=CARTESIAN_POINT('Ctrl Pts',(-0.573915184558107,-0.190326085855194,
0.795684265985088));
#6056=CARTESIAN_POINT('Ctrl Pts',(-0.548874290046456,-0.159766064500479,
0.813159949759));
#6057=CARTESIAN_POINT('Ctrl Pts',(-0.537715343527944,-0.142345102874864,
0.820511285096538));
#6058=CARTESIAN_POINT('Ctrl Pts',(-0.517157748491652,-0.0999305678883309,
0.833661031856294));
#6059=CARTESIAN_POINT('Ctrl Pts',(-0.508899795931835,-0.0740444353928835,
0.838633903678357));
#6060=CARTESIAN_POINT('Ctrl Pts',(-0.504455939115716,-0.04763,0.841298510752801));
#6061=CARTESIAN_POINT('Origin',(-0.707106781186548,-0.04763,0.707106781186547));
#6062=CARTESIAN_POINT('Origin',(0.,-0.04763,0.));
#6063=CARTESIAN_POINT('',(-0.951592097314,-0.04763,0.238183666596899));
#6064=CARTESIAN_POINT('Origin',(0.,-0.04763,0.));
#6065=CARTESIAN_POINT('Origin',(-1.,-0.04763,-1.11022302462516E-16));
#6066=CARTESIAN_POINT('Origin',(-1.,0.,-1.11022302462516E-16));
#6067=CARTESIAN_POINT('',(-0.951592097314,-0.04763,-0.2381836665969));
#6068=CARTESIAN_POINT('',(-0.980948,-0.246942143572133,1.08514323328844E-18));
#6069=CARTESIAN_POINT('Ctrl Pts',(-0.951592097314,-0.04763,-0.238183666596899));
#6070=CARTESIAN_POINT('Ctrl Pts',(-0.952850216871763,-0.0740444353928835,
-0.233157223576062));
#6071=CARTESIAN_POINT('Ctrl Pts',(-0.955173119738174,-0.0999305678883309,
-0.223801617934946));
#6072=CARTESIAN_POINT('Ctrl Pts',(-0.960411259488514,-0.142345102874864,
-0.199966927975188));
#6073=CARTESIAN_POINT('Ctrl Pts',(-0.963103647174702,-0.159766064500479,
-0.1868781821531));
#6074=CARTESIAN_POINT('Ctrl Pts',(-0.968453058988463,-0.190326085855194,
-0.15681442133453));
#6075=CARTESIAN_POINT('Ctrl Pts',(-0.971100730005489,-0.203463743702801,
-0.139836317888043));
#6076=CARTESIAN_POINT('Ctrl Pts',(-0.975530745318961,-0.224161999508995,
-0.104422493053067));
#6077=CARTESIAN_POINT('Ctrl Pts',(-0.977553872336861,-0.232861760990032,
-0.0842175114474175));
#6078=CARTESIAN_POINT('Ctrl Pts',(-0.980270995488453,-0.244251601209411,
-0.0421062857595699));
#6079=CARTESIAN_POINT('Ctrl Pts',(-0.980948,-0.246942143572133,-0.0201990724523195));
#6080=CARTESIAN_POINT('Ctrl Pts',(-0.980948,-0.246942143572133,-1.17961196366423E-16));
#6081=CARTESIAN_POINT('Origin',(-1.,-0.04763,-1.11022302462516E-16));
#6082=CARTESIAN_POINT('Ctrl Pts',(-0.980948,-0.246942143572133,-1.17961196366423E-16));
#6083=CARTESIAN_POINT('Ctrl Pts',(-0.980948,-0.246942143572133,0.0201990724523192));
#6084=CARTESIAN_POINT('Ctrl Pts',(-0.980270995488453,-0.244251601209411,
0.0421062857595695));
#6085=CARTESIAN_POINT('Ctrl Pts',(-0.977553872336861,-0.232861760990032,
0.0842175114474169));
#6086=CARTESIAN_POINT('Ctrl Pts',(-0.975530745318961,-0.224161999508995,
0.104422493053066));
#6087=CARTESIAN_POINT('Ctrl Pts',(-0.971100730005489,-0.203463743702801,
0.139836317888042));
#6088=CARTESIAN_POINT('Ctrl Pts',(-0.968453058988463,-0.190326085855194,
0.15681442133453));
#6089=CARTESIAN_POINT('Ctrl Pts',(-0.963103647174702,-0.15976606450048,
0.1868781821531));
#6090=CARTESIAN_POINT('Ctrl Pts',(-0.960411259488514,-0.142345102874864,
0.199966927975188));
#6091=CARTESIAN_POINT('Ctrl Pts',(-0.955173119738174,-0.099930567888331,
0.223801617934945));
#6092=CARTESIAN_POINT('Ctrl Pts',(-0.952850216871763,-0.0740444353928835,
0.233157223576061));
#6093=CARTESIAN_POINT('Ctrl Pts',(-0.951592097314,-0.04763,0.238183666596899));
#6094=CARTESIAN_POINT('Origin',(0.,-0.04763,0.));
#6095=CARTESIAN_POINT('',(-0.841298510752802,-0.04763,-0.504455939115715));
#6096=CARTESIAN_POINT('Origin',(0.,-0.04763,0.));
#6097=CARTESIAN_POINT('Origin',(-0.707106781186547,-0.04763,-0.707106781186548));
#6098=CARTESIAN_POINT('Origin',(-0.707106781186547,0.,-0.707106781186548));
#6099=CARTESIAN_POINT('',(-0.504455939115715,-0.04763,-0.841298510752802));
#6100=CARTESIAN_POINT('Ctrl Pts',(-0.504455939115715,-0.04763,-0.841298510752802));
#6101=CARTESIAN_POINT('Ctrl Pts',(-0.508899795931835,-0.0740444353928835,
-0.838633903678357));
#6102=CARTESIAN_POINT('Ctrl Pts',(-0.517157748491652,-0.0999305678883309,
-0.833661031856294));
#6103=CARTESIAN_POINT('Ctrl Pts',(-0.537715343527944,-0.142345102874864,
-0.820511285096538));
#6104=CARTESIAN_POINT('Ctrl Pts',(-0.548874290046456,-0.159766064500479,
-0.813159949759));
#6105=CARTESIAN_POINT('Ctrl Pts',(-0.573915184558107,-0.190326085855194,
-0.795684265985089));
#6106=CARTESIAN_POINT('Ctrl Pts',(-0.587792702767295,-0.203463743702801,
-0.78555112003688));
#6107=CARTESIAN_POINT('Ctrl Pts',(-0.615966552324775,-0.224161999508995,
-0.763642258217233));
#6108=CARTESIAN_POINT('Ctrl Pts',(-0.631684198665438,-0.232861760990032,
-0.750785745543687));
#6109=CARTESIAN_POINT('Ctrl Pts',(-0.663382628119203,-0.244251601209411,
-0.722929908501543));
#6110=CARTESIAN_POINT('Ctrl Pts',(-0.679352081686668,-0.246942143572133,
-0.707917883896095));
#6111=CARTESIAN_POINT('Ctrl Pts',(-0.707917883896095,-0.246942143572133,
-0.679352081686668));
#6112=CARTESIAN_POINT('Ctrl Pts',(-0.722929908501543,-0.244251601209411,
-0.663382628119203));
#6113=CARTESIAN_POINT('Ctrl Pts',(-0.750785745543687,-0.232861760990032,
-0.631684198665439));
#6114=CARTESIAN_POINT('Ctrl Pts',(-0.763642258217232,-0.224161999508995,
-0.615966552324775));
#6115=CARTESIAN_POINT('Ctrl Pts',(-0.78555112003688,-0.203463743702801,
-0.587792702767295));
#6116=CARTESIAN_POINT('Ctrl Pts',(-0.795684265985088,-0.190326085855194,
-0.573915184558107));
#6117=CARTESIAN_POINT('Ctrl Pts',(-0.813159949759,-0.15976606450048,-0.548874290046456));
#6118=CARTESIAN_POINT('Ctrl Pts',(-0.820511285096538,-0.142345102874864,
-0.537715343527944));
#6119=CARTESIAN_POINT('Ctrl Pts',(-0.833661031856294,-0.0999305678883311,
-0.517157748491652));
#6120=CARTESIAN_POINT('Ctrl Pts',(-0.838633903678357,-0.0740444353928836,
-0.508899795931835));
#6121=CARTESIAN_POINT('Ctrl Pts',(-0.841298510752801,-0.04763,-0.504455939115715));
#6122=CARTESIAN_POINT('Origin',(-0.707106781186547,-0.04763,-0.707106781186548));
#6123=CARTESIAN_POINT('Origin',(0.,-0.04763,0.));
#6124=CARTESIAN_POINT('',(-0.238183666596899,-0.04763,-0.951592097314));
#6125=CARTESIAN_POINT('Origin',(0.,-0.04763,0.));
#6126=CARTESIAN_POINT('Origin',(5.55111512312578E-17,-0.04763,-1.));
#6127=CARTESIAN_POINT('Origin',(5.55111512312578E-17,0.,-1.));
#6128=CARTESIAN_POINT('',(0.238183666596899,-0.04763,-0.951592097314));
#6129=CARTESIAN_POINT('Ctrl Pts',(0.238183666596899,-0.04763,-0.951592097314));
#6130=CARTESIAN_POINT('Ctrl Pts',(0.233157223576062,-0.0740444353928835,
-0.952850216871763));
#6131=CARTESIAN_POINT('Ctrl Pts',(0.223801617934946,-0.099930567888331,
-0.955173119738174));
#6132=CARTESIAN_POINT('Ctrl Pts',(0.199966927975188,-0.142345102874864,
-0.960411259488514));
#6133=CARTESIAN_POINT('Ctrl Pts',(0.1868781821531,-0.15976606450048,-0.963103647174702));
#6134=CARTESIAN_POINT('Ctrl Pts',(0.15681442133453,-0.190326085855194,-0.968453058988463));
#6135=CARTESIAN_POINT('Ctrl Pts',(0.139836317888042,-0.203463743702801,
-0.971100730005489));
#6136=CARTESIAN_POINT('Ctrl Pts',(0.104422493053067,-0.224161999508995,
-0.975530745318961));
#6137=CARTESIAN_POINT('Ctrl Pts',(0.0842175114474173,-0.232861760990032,
-0.977553872336861));
#6138=CARTESIAN_POINT('Ctrl Pts',(0.0421062857595698,-0.244251601209411,
-0.980270995488453));
#6139=CARTESIAN_POINT('Ctrl Pts',(0.0201990724523194,-0.246942143572133,
-0.980948));
#6140=CARTESIAN_POINT('Ctrl Pts',(-0.0201990724523193,-0.246942143572133,
-0.980948));
#6141=CARTESIAN_POINT('Ctrl Pts',(-0.0421062857595697,-0.244251601209411,
-0.980270995488453));
#6142=CARTESIAN_POINT('Ctrl Pts',(-0.0842175114474171,-0.232861760990032,
-0.977553872336861));
#6143=CARTESIAN_POINT('Ctrl Pts',(-0.104422493053067,-0.224161999508995,
-0.975530745318961));
#6144=CARTESIAN_POINT('Ctrl Pts',(-0.139836317888042,-0.203463743702801,
-0.971100730005489));
#6145=CARTESIAN_POINT('Ctrl Pts',(-0.15681442133453,-0.190326085855194,
-0.968453058988463));
#6146=CARTESIAN_POINT('Ctrl Pts',(-0.1868781821531,-0.15976606450048,-0.963103647174702));
#6147=CARTESIAN_POINT('Ctrl Pts',(-0.199966927975188,-0.142345102874864,
-0.960411259488514));
#6148=CARTESIAN_POINT('Ctrl Pts',(-0.223801617934945,-0.099930567888331,
-0.955173119738174));
#6149=CARTESIAN_POINT('Ctrl Pts',(-0.233157223576062,-0.0740444353928835,
-0.952850216871763));
#6150=CARTESIAN_POINT('Ctrl Pts',(-0.238183666596899,-0.0476299999999999,
-0.951592097314));
#6151=CARTESIAN_POINT('Origin',(5.55111512312578E-17,-0.04763,-1.));
#6152=CARTESIAN_POINT('Origin',(0.,-0.04763,0.));
#6153=CARTESIAN_POINT('',(0.504455939115715,-0.04763,-0.841298510752802));
#6154=CARTESIAN_POINT('Origin',(0.,-0.04763,0.));
#6155=CARTESIAN_POINT('Origin',(0.707106781186548,-0.04763,-0.707106781186547));
#6156=CARTESIAN_POINT('Origin',(0.707106781186548,0.,-0.707106781186547));
#6157=CARTESIAN_POINT('',(0.841298510752802,-0.04763,-0.504455939115715));
#6158=CARTESIAN_POINT('Ctrl Pts',(0.841298510752802,-0.04763,-0.504455939115715));
#6159=CARTESIAN_POINT('Ctrl Pts',(0.838633903678357,-0.0740444353928835,
-0.508899795931835));
#6160=CARTESIAN_POINT('Ctrl Pts',(0.833661031856294,-0.0999305678883309,
-0.517157748491652));
#6161=CARTESIAN_POINT('Ctrl Pts',(0.820511285096538,-0.142345102874864,
-0.537715343527944));
#6162=CARTESIAN_POINT('Ctrl Pts',(0.813159949759,-0.159766064500479,-0.548874290046456));
#6163=CARTESIAN_POINT('Ctrl Pts',(0.795684265985088,-0.190326085855194,
-0.573915184558107));
#6164=CARTESIAN_POINT('Ctrl Pts',(0.78555112003688,-0.203463743702801,-0.587792702767295));
#6165=CARTESIAN_POINT('Ctrl Pts',(0.763642258217233,-0.224161999508995,
-0.615966552324775));
#6166=CARTESIAN_POINT('Ctrl Pts',(0.750785745543687,-0.232861760990032,
-0.631684198665438));
#6167=CARTESIAN_POINT('Ctrl Pts',(0.722929908501543,-0.244251601209411,
-0.663382628119203));
#6168=CARTESIAN_POINT('Ctrl Pts',(0.707917883896095,-0.246942143572133,
-0.679352081686668));
#6169=CARTESIAN_POINT('Ctrl Pts',(0.679352081686668,-0.246942143572133,
-0.707917883896095));
#6170=CARTESIAN_POINT('Ctrl Pts',(0.663382628119203,-0.244251601209411,
-0.722929908501543));
#6171=CARTESIAN_POINT('Ctrl Pts',(0.631684198665438,-0.232861760990032,
-0.750785745543687));
#6172=CARTESIAN_POINT('Ctrl Pts',(0.615966552324775,-0.224161999508995,
-0.763642258217232));
#6173=CARTESIAN_POINT('Ctrl Pts',(0.587792702767295,-0.203463743702801,
-0.78555112003688));
#6174=CARTESIAN_POINT('Ctrl Pts',(0.573915184558107,-0.190326085855194,
-0.795684265985088));
#6175=CARTESIAN_POINT('Ctrl Pts',(0.548874290046456,-0.159766064500479,
-0.813159949759));
#6176=CARTESIAN_POINT('Ctrl Pts',(0.537715343527944,-0.142345102874864,
-0.820511285096538));
#6177=CARTESIAN_POINT('Ctrl Pts',(0.517157748491652,-0.099930567888331,
-0.833661031856294));
#6178=CARTESIAN_POINT('Ctrl Pts',(0.508899795931835,-0.0740444353928835,
-0.838633903678357));
#6179=CARTESIAN_POINT('Ctrl Pts',(0.504455939115715,-0.04763,-0.841298510752801));
#6180=CARTESIAN_POINT('Origin',(0.707106781186548,-0.04763,-0.707106781186547));
#6181=CARTESIAN_POINT('Origin',(0.,-0.166705,0.));
#6182=CARTESIAN_POINT('',(-0.980948,-0.28578,1.20131482833E-16));
#6183=CARTESIAN_POINT('Origin',(0.,-0.28578,0.));
#6184=CARTESIAN_POINT('',(-0.980948,-0.166705,1.20131482833E-16));
#6185=CARTESIAN_POINT('',(0.951592097314,-0.04763,0.238183666596899));
#6186=CARTESIAN_POINT('Origin',(0.,-0.04763,0.));
#6187=CARTESIAN_POINT('',(0.951592097314,-0.04763,-0.238183666596899));
#6188=CARTESIAN_POINT('Ctrl Pts',(0.951592097314,-0.04763,0.238183666596899));
#6189=CARTESIAN_POINT('Ctrl Pts',(0.952850216871763,-0.0740444353928835,
0.233157223576062));
#6190=CARTESIAN_POINT('Ctrl Pts',(0.955173119738174,-0.099930567888331,
0.223801617934945));
#6191=CARTESIAN_POINT('Ctrl Pts',(0.960411259488514,-0.142345102874864,
0.199966927975188));
#6192=CARTESIAN_POINT('Ctrl Pts',(0.963103647174702,-0.15976606450048,0.1868781821531));
#6193=CARTESIAN_POINT('Ctrl Pts',(0.968453058988463,-0.190326085855194,
0.15681442133453));
#6194=CARTESIAN_POINT('Ctrl Pts',(0.971100730005489,-0.203463743702801,
0.139836317888042));
#6195=CARTESIAN_POINT('Ctrl Pts',(0.975530745318961,-0.224161999508995,
0.104422493053067));
#6196=CARTESIAN_POINT('Ctrl Pts',(0.977553872336861,-0.232861760990032,
0.0842175114474172));
#6197=CARTESIAN_POINT('Ctrl Pts',(0.980270995488453,-0.244251601209411,
0.0421062857595697));
#6198=CARTESIAN_POINT('Ctrl Pts',(0.980948,-0.246942143572133,0.0201990724523194));
#6199=CARTESIAN_POINT('Ctrl Pts',(0.980948,-0.246942143572133,-0.0201990724523194));
#6200=CARTESIAN_POINT('Ctrl Pts',(0.980270995488453,-0.244251601209411,
-0.0421062857595697));
#6201=CARTESIAN_POINT('Ctrl Pts',(0.977553872336861,-0.232861760990032,
-0.0842175114474172));
#6202=CARTESIAN_POINT('Ctrl Pts',(0.975530745318961,-0.224161999508995,
-0.104422493053067));
#6203=CARTESIAN_POINT('Ctrl Pts',(0.971100730005489,-0.203463743702801,
-0.139836317888042));
#6204=CARTESIAN_POINT('Ctrl Pts',(0.968453058988463,-0.190326085855194,
-0.15681442133453));
#6205=CARTESIAN_POINT('Ctrl Pts',(0.963103647174702,-0.15976606450048,-0.1868781821531));
#6206=CARTESIAN_POINT('Ctrl Pts',(0.960411259488514,-0.142345102874864,
-0.199966927975188));
#6207=CARTESIAN_POINT('Ctrl Pts',(0.955173119738174,-0.099930567888331,
-0.223801617934945));
#6208=CARTESIAN_POINT('Ctrl Pts',(0.952850216871763,-0.0740444353928835,
-0.233157223576062));
#6209=CARTESIAN_POINT('Ctrl Pts',(0.951592097314,-0.0476299999999999,-0.238183666596899));
#6210=CARTESIAN_POINT('Origin',(0.,-0.04763,0.));
#6211=CARTESIAN_POINT('Origin',(0.,-0.04763,0.));
#6212=CARTESIAN_POINT('Origin',(1.,-0.04763,0.));
#6213=CARTESIAN_POINT('Origin',(1.,0.,0.));
#6214=CARTESIAN_POINT('Origin',(1.,-0.04763,0.));
#6215=CARTESIAN_POINT('Origin',(0.,-0.28578,0.));
#6216=CARTESIAN_POINT('Origin',(0.,-0.04763,0.));
#6674=UNCERTAINTY_MEASURE_WITH_UNIT(LENGTH_MEASURE(0.001),#6706,
'DISTANCE_ACCURACY_VALUE',
'Maximum model space distance between geometric entities at asserted c
onnectivities');
#6683=UNCERTAINTY_MEASURE_WITH_UNIT(LENGTH_MEASURE(0.001),#6706,
'DISTANCE_ACCURACY_VALUE',
'Maximum model space distance between geometric entities at asserted c
onnectivities');
#6696=(
GEOMETRIC_REPRESENTATION_CONTEXT(3)
GLOBAL_UNCERTAINTY_ASSIGNED_CONTEXT((#6674))
GLOBAL_UNIT_ASSIGNED_CONTEXT((#6706,#6708,#6709))
REPRESENTATION_CONTEXT('','3D')
);
#6705=(
GEOMETRIC_REPRESENTATION_CONTEXT(3)
GLOBAL_UNCERTAINTY_ASSIGNED_CONTEXT((#6683))
GLOBAL_UNIT_ASSIGNED_CONTEXT((#6706,#6708,#6709))
REPRESENTATION_CONTEXT('','3D')
);
#6706=(
LENGTH_UNIT()
NAMED_UNIT(*)
SI_UNIT(.CENTI.,.METRE.)
);
#6708=(
NAMED_UNIT(*)
PLANE_ANGLE_UNIT()
SI_UNIT($,.RADIAN.)
);
#6709=(
NAMED_UNIT(*)
SI_UNIT($,.STERADIAN.)
SOLID_ANGLE_UNIT()
);
#6722=SHAPE_DEFINITION_REPRESENTATION(#6743,#6823);
#6743=PRODUCT_DEFINITION_SHAPE('',$,#6845);
#6823=SHAPE_REPRESENTATION('',(#3805),#6696);
#6832=PRODUCT_DEFINITION_CONTEXT('part definition',#6897,'design');
#6845=PRODUCT_DEFINITION('Cage','Cage',#6866,#6832);
#6866=PRODUCT_DEFINITION_FORMATION('',$,#6911);
#6897=APPLICATION_CONTEXT(
'Core Data for Automotive Mechanical Design Process');
#6898=PRODUCT_CONTEXT('part definition',#6897,'mechanical');
#6911=PRODUCT('Cage','Cage','Cage',(#6898));
#6983=COLOUR_RGB('Grey',0.48,0.52,0.57);
#6984=FILL_AREA_STYLE_COLOUR('',#6983);
#6985=FILL_AREA_STYLE('',(#6984));
#6986=SURFACE_STYLE_FILL_AREA(#6985);
#6987=SURFACE_SIDE_STYLE('',(#6986));
#6988=SURFACE_STYLE_USAGE(.BOTH.,#6987);
#6989=PRESENTATION_STYLE_ASSIGNMENT((#6988));
ENDSEC;
END-ISO-10303-21;
